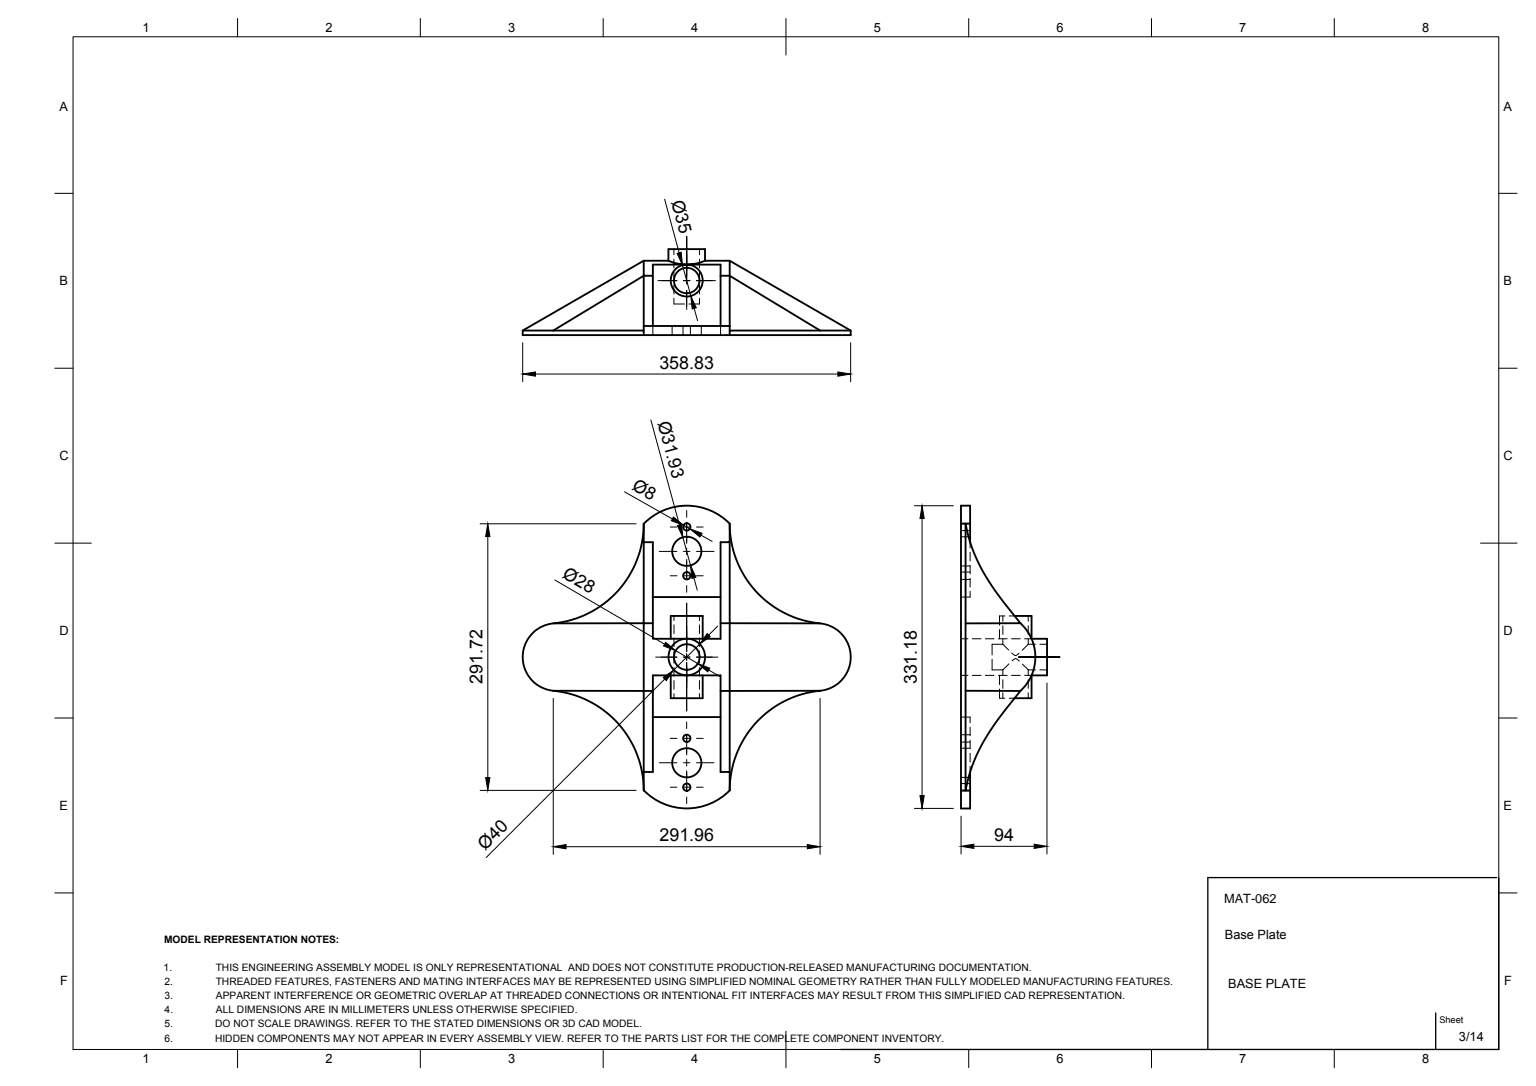
ISO-10303-21;
HEADER;
/* Generated by software containing ST-Developer
 * from STEP Tools, Inc. (www.steptools.com) 
 */

FILE_DESCRIPTION(
/* description */ (''),
/* implementation_level */ '2;1');

FILE_NAME(
/* name */ 'Base Plate.step',
/* time_stamp */ '2026-10-24T10:18:25-07:00',
/* author */ (''),
/* organization */ (''),
/* preprocessor_version */ 'ST-DEVELOPER v20.2',
/* originating_system */ 'Autodesk Translation Framework v15.15.0.0',
/* authorisation */ '');

FILE_SCHEMA (('AUTOMOTIVE_DESIGN { 1 0 10303 214 3 1 1 }'));
ENDSEC;

DATA;
#10=MECHANICAL_DESIGN_GEOMETRIC_PRESENTATION_REPRESENTATION('',(#247),#14125);
#227=SHAPE_REPRESENTATION_RELATIONSHIP('SRR','None',#14200,#237);
#237=ADVANCED_BREP_SHAPE_REPRESENTATION('',(#266),#14114);
#247=STYLED_ITEM('',(#14263),#266);
#266=MANIFOLD_SOLID_BREP('Base Plate',#6134);
#279=B_SPLINE_SURFACE_WITH_KNOTS('',3,1,((#9488,#9489),(#9490,#9491),(#9492,
#9493),(#9494,#9495),(#9496,#9497),(#9498,#9499),(#9500,#9501),(#9502,#9503),
(#9504,#9505),(#9506,#9507),(#9508,#9509),(#9510,#9511),(#9512,#9513),(#9514,
#9515),(#9516,#9517),(#9518,#9519),(#9520,#9521),(#9522,#9523),(#9524,#9525),
(#9526,#9527),(#9528,#9529),(#9530,#9531),(#9532,#9533),(#9534,#9535),(#9536,
#9537),(#9538,#9539),(#9540,#9541),(#9542,#9543),(#9544,#9545),(#9546,#9547)),
 .UNSPECIFIED.,.F.,.F.,.F.,(4,2,2,2,2,2,2,2,2,2,2,2,2,2,4),(2,2),(0.,0.125000000000001,
0.1875,0.25,0.3125,0.375,0.4375,0.5,0.5625,0.625,0.6875,0.75,0.8125,0.875,
1.),(0.,1.00875859451262),.UNSPECIFIED.);
#280=B_SPLINE_SURFACE_WITH_KNOTS('',3,1,((#9560,#9561),(#9562,#9563),(#9564,
#9565),(#9566,#9567),(#9568,#9569),(#9570,#9571),(#9572,#9573),(#9574,#9575),
(#9576,#9577),(#9578,#9579),(#9580,#9581),(#9582,#9583),(#9584,#9585),(#9586,
#9587),(#9588,#9589),(#9590,#9591),(#9592,#9593),(#9594,#9595),(#9596,#9597),
(#9598,#9599),(#9600,#9601),(#9602,#9603),(#9604,#9605),(#9606,#9607),(#9608,
#9609),(#9610,#9611),(#9612,#9613),(#9614,#9615),(#9616,#9617),(#9618,#9619)),
 .UNSPECIFIED.,.F.,.F.,.F.,(4,2,2,2,2,2,2,2,2,2,2,2,2,2,4),(2,2),(0.,0.125,
0.1875,0.25,0.312499999999999,0.374999999999999,0.437499999999999,0.499999999999999,
0.562499999999999,0.624999999999999,0.687499999999999,0.75,0.8125,0.875,
1.),(0.,1.00875859529089),.UNSPECIFIED.);
#281=B_SPLINE_SURFACE_WITH_KNOTS('',3,1,((#9630,#9631),(#9632,#9633),(#9634,
#9635),(#9636,#9637),(#9638,#9639),(#9640,#9641),(#9642,#9643),(#9644,#9645),
(#9646,#9647),(#9648,#9649),(#9650,#9651),(#9652,#9653),(#9654,#9655),(#9656,
#9657),(#9658,#9659),(#9660,#9661),(#9662,#9663),(#9664,#9665),(#9666,#9667),
(#9668,#9669),(#9670,#9671),(#9672,#9673),(#9674,#9675),(#9676,#9677),(#9678,
#9679),(#9680,#9681),(#9682,#9683),(#9684,#9685),(#9686,#9687),(#9688,#9689),
(#9690,#9691),(#9692,#9693),(#9694,#9695),(#9696,#9697)),.UNSPECIFIED.,
 .F.,.F.,.F.,(4,2,2,2,2,2,2,2,2,2,2,2,2,2,2,2,4),(2,2),(0.,0.0625,0.125,
0.1875,0.25,0.3125,0.375,0.4375,0.5,0.5625,0.625,0.6875,0.75,0.8125,0.875,
0.9375,1.),(0.,1.),.UNSPECIFIED.);
#282=B_SPLINE_SURFACE_WITH_KNOTS('',3,1,((#9723,#9724),(#9725,#9726),(#9727,
#9728),(#9729,#9730)),.UNSPECIFIED.,.F.,.F.,.F.,(4,4),(2,2),(0.14457615148808,
1.),(0.,1.2),.UNSPECIFIED.);
#283=B_SPLINE_SURFACE_WITH_KNOTS('',3,1,((#9770,#9771),(#9772,#9773),(#9774,
#9775),(#9776,#9777)),.UNSPECIFIED.,.F.,.F.,.F.,(4,4),(2,2),(0.,0.855423965834485),
(0.,1.2),.UNSPECIFIED.);
#284=B_SPLINE_SURFACE_WITH_KNOTS('',3,1,((#9934,#9935),(#9936,#9937),(#9938,
#9939),(#9940,#9941),(#9942,#9943),(#9944,#9945),(#9946,#9947),(#9948,#9949),
(#9950,#9951),(#9952,#9953),(#9954,#9955),(#9956,#9957),(#9958,#9959),(#9960,
#9961),(#9962,#9963),(#9964,#9965),(#9966,#9967),(#9968,#9969),(#9970,#9971),
(#9972,#9973),(#9974,#9975),(#9976,#9977),(#9978,#9979),(#9980,#9981),(#9982,
#9983),(#9984,#9985),(#9986,#9987),(#9988,#9989),(#9990,#9991),(#9992,#9993)),
 .UNSPECIFIED.,.F.,.F.,.F.,(4,2,2,2,2,2,2,2,2,2,2,2,2,2,4),(2,2),(0.,0.125000000000001,
0.1875,0.25,0.3125,0.375,0.4375,0.5,0.5625,0.625,0.6875,0.75,0.8125,0.875,
1.),(0.,1.00875859388372),.UNSPECIFIED.);
#285=B_SPLINE_SURFACE_WITH_KNOTS('',3,1,((#9999,#10000),(#10001,#10002),
(#10003,#10004),(#10005,#10006),(#10007,#10008),(#10009,#10010),(#10011,
#10012),(#10013,#10014),(#10015,#10016),(#10017,#10018),(#10019,#10020),
(#10021,#10022),(#10023,#10024),(#10025,#10026),(#10027,#10028),(#10029,
#10030),(#10031,#10032),(#10033,#10034),(#10035,#10036),(#10037,#10038),
(#10039,#10040),(#10041,#10042),(#10043,#10044),(#10045,#10046),(#10047,
#10048),(#10049,#10050),(#10051,#10052),(#10053,#10054),(#10055,#10056),
(#10057,#10058)),.UNSPECIFIED.,.F.,.F.,.F.,(4,2,2,2,2,2,2,2,2,2,2,2,2,2,
4),(2,2),(0.,0.125,0.1875,0.25,0.312499999999999,0.374999999999999,0.437499999999999,
0.499999999999999,0.562499999999999,0.624999999999999,0.687499999999999,
0.75,0.8125,0.875,1.),(0.,1.00875859641008),.UNSPECIFIED.);
#286=B_SPLINE_SURFACE_WITH_KNOTS('',3,1,((#10064,#10065),(#10066,#10067),
(#10068,#10069),(#10070,#10071),(#10072,#10073),(#10074,#10075),(#10076,
#10077),(#10078,#10079),(#10080,#10081),(#10082,#10083),(#10084,#10085),
(#10086,#10087),(#10088,#10089),(#10090,#10091),(#10092,#10093),(#10094,
#10095),(#10096,#10097),(#10098,#10099),(#10100,#10101),(#10102,#10103),
(#10104,#10105),(#10106,#10107),(#10108,#10109),(#10110,#10111),(#10112,
#10113),(#10114,#10115),(#10116,#10117),(#10118,#10119),(#10120,#10121),
(#10122,#10123),(#10124,#10125),(#10126,#10127),(#10128,#10129),(#10130,
#10131)),.UNSPECIFIED.,.F.,.F.,.F.,(4,2,2,2,2,2,2,2,2,2,2,2,2,2,2,2,4),
(2,2),(0.,0.0625,0.125,0.1875,0.25,0.3125,0.375,0.4375,0.5,0.5625,0.625,
0.6875,0.75,0.8125,0.875,0.9375,1.),(0.,1.),.UNSPECIFIED.);
#287=B_SPLINE_SURFACE_WITH_KNOTS('',3,1,((#10132,#10133),(#10134,#10135),
(#10136,#10137),(#10138,#10139)),.UNSPECIFIED.,.F.,.F.,.F.,(4,4),(2,2),
(0.144576151499063,1.),(0.,1.20000000000001),.UNSPECIFIED.);
#288=B_SPLINE_SURFACE_WITH_KNOTS('',3,1,((#10140,#10141),(#10142,#10143),
(#10144,#10145),(#10146,#10147)),.UNSPECIFIED.,.F.,.F.,.F.,(4,4),(2,2),
(0.,0.855423965822116),(0.,1.2),.UNSPECIFIED.);
#292=B_SPLINE_CURVE_WITH_KNOTS('',3,(#8671,#8672,#8673,#8674,#8675,#8676,
#8677,#8678,#8679,#8680,#8681,#8682,#8683,#8684,#8685,#8686,#8687,#8688,
#8689,#8690,#8691,#8692,#8693,#8694,#8695,#8696,#8697,#8698,#8699,#8700,
#8701,#8702,#8703,#8704,#8705,#8706,#8707,#8708),.UNSPECIFIED.,.F.,.F.,
(4,2,2,2,2,2,2,2,2,2,2,2,2,2,2,2,2,2,4),(0.,0.0927340025111304,0.185468005022261,
0.370936010044522,0.741872020089043,1.11280803013356,1.48374404017809,2.05783904851561,
2.34488655268438,2.63193405685314,2.9189815610219,3.20602906519066,3.78012407352819,
4.15106008357271,4.52199609361724,4.89293210366176,5.07840010868402,5.17113411119515,
5.26386811370629),.UNSPECIFIED.);
#293=B_SPLINE_CURVE_WITH_KNOTS('',3,(#8709,#8710,#8711,#8712,#8713,#8714,
#8715,#8716,#8717,#8718,#8719,#8720,#8721,#8722,#8723,#8724,#8725,#8726,
#8727,#8728,#8729,#8730,#8731,#8732,#8733,#8734,#8735,#8736,#8737,#8738,
#8739,#8740,#8741,#8742,#8743,#8744,#8745,#8746),.UNSPECIFIED.,.F.,.F.,
(4,2,2,2,2,2,2,2,2,2,2,2,2,2,2,2,2,2,4),(5.26386811370629,5.35660211621742,
5.44933611872855,5.63480412375081,6.00574013379534,6.37667614383986,6.74761215388439,
7.32170716222191,7.60875466639068,7.89580217055944,8.1828496747282,8.46989717889697,
9.0439921872345,9.41492819727902,9.78586420732354,10.1568002173681,10.3422682223903,
10.4350022249015,10.5277362274126),.UNSPECIFIED.);
#294=B_SPLINE_CURVE_WITH_KNOTS('',3,(#8749,#8750,#8751,#8752,#8753,#8754,
#8755,#8756,#8757,#8758,#8759,#8760,#8761,#8762,#8763,#8764,#8765,#8766,
#8767,#8768,#8769,#8770,#8771,#8772,#8773,#8774,#8775,#8776,#8777,#8778,
#8779,#8780,#8781,#8782,#8783,#8784,#8785,#8786),.UNSPECIFIED.,.F.,.F.,
(4,2,2,2,2,2,2,2,2,2,2,2,2,2,2,2,2,2,4),(0.,0.0927340025111308,0.185468005022262,
0.370936010044523,0.741872020089046,1.11280803013357,1.48374404017809,2.05783904851562,
2.34488655268438,2.63193405685315,2.91898156102191,3.20602906519068,3.7801240735282,
4.15106008357273,4.52199609361725,4.89293210366178,5.07840010868404,5.17113411119517,
5.2638681137063),.UNSPECIFIED.);
#295=B_SPLINE_CURVE_WITH_KNOTS('',3,(#8787,#8788,#8789,#8790,#8791,#8792,
#8793,#8794,#8795,#8796,#8797,#8798,#8799,#8800,#8801,#8802,#8803,#8804,
#8805,#8806,#8807,#8808,#8809,#8810,#8811,#8812,#8813,#8814,#8815,#8816,
#8817,#8818,#8819,#8820,#8821,#8822,#8823,#8824),.UNSPECIFIED.,.F.,.F.,
(4,2,2,2,2,2,2,2,2,2,2,2,2,2,2,2,2,2,4),(5.2638681137063,5.35660211621743,
5.44933611872857,5.63480412375083,6.00574013379535,6.37667614383987,6.7476121538844,
7.32170716222192,7.60875466639069,7.89580217055945,8.18284967472821,8.46989717889698,
9.0439921872345,9.41492819727902,9.78586420732355,10.1568002173681,10.3422682223903,
10.4350022249015,10.5277362274126),.UNSPECIFIED.);
#296=B_SPLINE_CURVE_WITH_KNOTS('',3,(#8834,#8835,#8836,#8837,#8838,#8839,
#8840,#8841,#8842,#8843,#8844,#8845,#8846,#8847,#8848,#8849,#8850,#8851),
 .UNSPECIFIED.,.F.,.F.,(4,2,2,2,2,2,2,2,4),(9.15255602234747,9.53372020064684,
9.91488437894621,10.2960485572456,10.6772127355449,11.0587615591079,11.4403103826708,
11.8218592062337,12.2034080297966),.UNSPECIFIED.);
#297=B_SPLINE_CURVE_WITH_KNOTS('',3,(#8853,#8854,#8855,#8856,#8857,#8858,
#8859,#8860,#8861,#8862,#8863,#8864,#8865,#8866,#8867,#8868,#8869,#8870),
 .UNSPECIFIED.,.F.,.F.,(4,2,2,2,2,2,2,2,4),(6.10170401489831,6.48325283846123,
6.86480166202415,7.24635048558707,7.62789930914999,8.00906348744936,8.39022766574873,
8.7713918440481,9.15255602234747),.UNSPECIFIED.);
#298=B_SPLINE_CURVE_WITH_KNOTS('',3,(#8878,#8879,#8880,#8881,#8882,#8883,
#8884,#8885,#8886,#8887,#8888,#8889,#8890,#8891,#8892,#8893,#8894,#8895,
#8896,#8897,#8898,#8899,#8900,#8901,#8902),.UNSPECIFIED.,.F.,.F.,(4,3,3,
3,3,3,3,3,4),(-1.,-0.875,-0.75,-0.625,-0.5,-0.375,-0.25,-0.125,0.),
 .UNSPECIFIED.);
#299=B_SPLINE_CURVE_WITH_KNOTS('',3,(#8935,#8936,#8937,#8938,#8939,#8940,
#8941,#8942,#8943,#8944,#8945,#8946,#8947,#8948,#8949,#8950,#8951,#8952,
#8953,#8954,#8955,#8956,#8957,#8958,#8959,#8960,#8961,#8962,#8963,#8964,
#8965,#8966,#8967,#8968,#8969,#8970,#8971,#8972,#8973,#8974,#8975,#8976,
#8977,#8978,#8979,#8980,#8981,#8982,#8983,#8984,#8985,#8986,#8987,#8988,
#8989,#8990,#8991,#8992,#8993,#8994,#8995,#8996,#8997,#8998,#8999,#9000,
#9001,#9002,#9003,#9004,#9005,#9006,#9007,#9008,#9009,#9010,#9011,#9012,
#9013,#9014,#9015,#9016,#9017,#9018,#9019,#9020,#9021,#9022,#9023,#9024,
#9025,#9026,#9027,#9028,#9029,#9030,#9031,#9032,#9033,#9034,#9035,#9036,
#9037,#9038,#9039,#9040,#9041,#9042,#9043,#9044,#9045,#9046,#9047,#9048,
#9049,#9050,#9051,#9052,#9053,#9054,#9055,#9056,#9057,#9058,#9059,#9060,
#9061,#9062,#9063,#9064,#9065,#9066,#9067,#9068,#9069,#9070,#9071,#9072,
#9073,#9074,#9075,#9076,#9077,#9078,#9079,#9080,#9081,#9082,#9083,#9084,
#9085,#9086,#9087,#9088,#9089,#9090,#9091,#9092,#9093,#9094,#9095,#9096,
#9097,#9098,#9099,#9100,#9101,#9102,#9103,#9104,#9105,#9106,#9107,#9108,
#9109,#9110,#9111,#9112,#9113,#9114,#9115,#9116,#9117,#9118),
 .UNSPECIFIED.,.F.,.F.,(4,3,3,3,3,3,3,3,3,3,3,3,3,3,3,3,3,3,3,3,3,3,3,3,
3,3,3,3,3,3,3,3,3,3,3,3,3,3,3,3,3,3,3,3,3,3,3,3,3,3,3,3,3,3,3,3,3,3,3,3,
3,4),(0.150241198747907,0.167397304835228,0.184718118887321,0.202241047709381,
0.220007464163269,0.238064286953153,0.24996953246951,0.25115288079109,0.277756413628116,
0.304952901732967,0.332851547605054,0.361595243786114,0.371570318101956,
0.374891379875467,0.37684512588001,0.404565053134646,0.433143322897528,
0.46278930680584,0.493811743368577,0.49776633912351,0.499650446210555,0.501139153619483,
0.526262386397414,0.552281259081706,0.580263680389099,0.606497200364781,
0.618794162853381,0.622041027561349,0.623773539268005,0.624868539292833,
0.62607780545653,0.662083917086729,0.720106829170489,0.737600152347333,
0.745800147586479,0.747905908951524,0.749388388026565,0.749955707873429,
0.750554094407055,0.771533017768898,0.793328350135385,0.806245328251924,
0.812300161744051,0.812901601299671,0.828591002192834,0.846067273157757,
0.865308864013037,0.873727060012223,0.874713567355877,0.87499463526931,
0.875252029008748,0.898077041623502,0.91317689673975,0.926104230971432,
0.935341202100003,0.937361789534378,0.937508712583833,0.949516479167898,
0.963001489246603,0.977729187677142,0.995717213427348,1.),.UNSPECIFIED.);
#300=B_SPLINE_CURVE_WITH_KNOTS('',3,(#9125,#9126,#9127,#9128,#9129,#9130,
#9131,#9132,#9133,#9134,#9135,#9136,#9137,#9138,#9139,#9140,#9141,#9142,
#9143,#9144,#9145,#9146,#9147,#9148,#9149,#9150,#9151,#9152,#9153,#9154,
#9155,#9156,#9157,#9158,#9159,#9160,#9161,#9162,#9163,#9164,#9165,#9166,
#9167,#9168,#9169,#9170,#9171,#9172,#9173,#9174,#9175,#9176,#9177,#9178,
#9179,#9180,#9181,#9182,#9183,#9184,#9185,#9186,#9187,#9188,#9189,#9190,
#9191,#9192,#9193,#9194,#9195,#9196,#9197,#9198,#9199,#9200,#9201,#9202,
#9203,#9204,#9205,#9206,#9207,#9208,#9209,#9210,#9211,#9212,#9213,#9214,
#9215,#9216,#9217,#9218,#9219,#9220,#9221,#9222,#9223,#9224,#9225,#9226,
#9227,#9228,#9229,#9230,#9231,#9232,#9233,#9234,#9235,#9236,#9237,#9238,
#9239,#9240,#9241,#9242,#9243,#9244,#9245,#9246,#9247,#9248,#9249,#9250,
#9251,#9252,#9253,#9254,#9255,#9256,#9257,#9258,#9259,#9260,#9261,#9262,
#9263,#9264,#9265,#9266,#9267,#9268,#9269,#9270,#9271,#9272,#9273,#9274,
#9275,#9276,#9277,#9278,#9279,#9280,#9281,#9282,#9283,#9284,#9285,#9286,
#9287,#9288,#9289,#9290,#9291,#9292,#9293,#9294,#9295,#9296,#9297,#9298,
#9299,#9300,#9301,#9302,#9303,#9304,#9305),.UNSPECIFIED.,.F.,.F.,(4,3,3,
3,3,3,3,3,3,3,3,3,3,3,3,3,3,3,3,3,3,3,3,3,3,3,3,3,3,3,3,3,3,3,3,3,3,3,3,
3,3,3,3,3,3,3,3,3,3,3,3,3,3,3,3,3,3,3,3,3,4),(0.,0.0173864418603424,0.0317406407068232,
0.0445735019151384,0.0571545623287322,0.0602506826648901,0.0617926957229375,
0.0622286000993027,0.0624303599347524,0.062594733958677,0.0746665408516836,
0.0885152798747999,0.106661753514485,0.118272684996839,0.12398744033581,
0.12469708287651,0.124978108020046,0.125243557342601,0.14788473893768,0.165674472900084,
0.181276305626835,0.186498845179634,0.187421439977098,0.188081999482287,
0.210113337373066,0.230102338342194,0.249466683031036,0.250074016598888,
0.290650259758732,0.333611006225432,0.365870403860414,0.373431200181113,
0.37495605866907,0.376045195512328,0.405652456316879,0.433409263321146,
0.459431269887646,0.483826901043739,0.495262353148158,0.498872802540326,
0.501065640438556,0.531952057906504,0.561479569871501,0.589959832895018,
0.617600948986098,0.624836289376345,0.626872446293665,0.655342990004338,
0.683068491132681,0.710166098531947,0.73672700441613,0.743791652164193,
0.747103205796098,0.748975108318689,0.750181999132194,0.768352317329036,
0.786243445752231,0.803790273865076,0.82117579398772,0.838357975229974,
0.849761368385144),.UNSPECIFIED.);
#301=B_SPLINE_CURVE_WITH_KNOTS('',3,(#9309,#9310,#9311,#9312),
 .UNSPECIFIED.,.F.,.F.,(4,4),(0.149678083001057,0.999999081493329),
 .UNSPECIFIED.);
#302=B_SPLINE_CURVE_WITH_KNOTS('',3,(#9316,#9317,#9318,#9319),
 .UNSPECIFIED.,.F.,.F.,(4,4),(1.03512807303671E-6,0.850322033620394),
 .UNSPECIFIED.);
#303=B_SPLINE_CURVE_WITH_KNOTS('',3,(#9322,#9323,#9324,#9325),
 .UNSPECIFIED.,.F.,.F.,(4,4),(-1.,-0.850320998496977),.UNSPECIFIED.);
#304=B_SPLINE_CURVE_WITH_KNOTS('',3,(#9330,#9331,#9332,#9333,#9334,#9335),
 .UNSPECIFIED.,.F.,.F.,(4,2,4),(0.,0.125000000000001,0.149679001503013),
 .UNSPECIFIED.);
#305=B_SPLINE_CURVE_WITH_KNOTS('',3,(#9339,#9340,#9341,#9342,#9343,#9344,
#9345,#9346,#9347,#9348,#9349,#9350,#9351,#9352,#9353,#9354,#9355,#9356,
#9357,#9358,#9359,#9360,#9361,#9362,#9363,#9364,#9365,#9366,#9367,#9368,
#9369,#9370,#9371,#9372,#9373,#9374,#9375,#9376,#9377,#9378,#9379,#9380,
#9381,#9382,#9383,#9384),.UNSPECIFIED.,.F.,.F.,(4,3,3,3,3,3,3,3,3,3,3,3,
3,3,3,4),(-16.2042554582664,-16.1371180260605,-14.2967993206844,-13.2982156828388,
-12.2761212402173,-11.2362598068131,-10.1850784450982,-9.12964303443693,
-8.07313766648818,-7.01663510715248,-5.96496475382742,-4.92301254140941,
-3.89517570042547,-2.88556286360814,-1.89741455218585,0.),.UNSPECIFIED.);
#306=B_SPLINE_CURVE_WITH_KNOTS('',3,(#9390,#9391,#9392,#9393,#9394,#9395,
#9396,#9397,#9398,#9399,#9400,#9401,#9402,#9403,#9404,#9405,#9406,#9407,
#9408,#9409,#9410,#9411,#9412,#9413,#9414,#9415,#9416,#9417,#9418,#9419,
#9420,#9421,#9422,#9423,#9424,#9425,#9426,#9427,#9428,#9429,#9430,#9431,
#9432,#9433,#9434,#9435),.UNSPECIFIED.,.F.,.F.,(4,3,3,3,3,3,3,3,3,3,3,3,
3,3,3,4),(-0.0671460795128853,0.,1.84055573902674,2.83926799475898,3.86149408346386,
4.90148945134311,5.95280620554087,7.00837755660534,8.06501900276707,9.12165763995372,
10.1734634487402,11.2155498649205,12.2435190916037,13.2532619668624,14.2415375520883,
16.1391964918471),.UNSPECIFIED.);
#307=B_SPLINE_CURVE_WITH_KNOTS('',3,(#9439,#9440,#9441,#9442,#9443,#9444,
#9445,#9446,#9447,#9448,#9449,#9450,#9451,#9452,#9453,#9454,#9455,#9456,
#9457,#9458,#9459,#9460,#9461,#9462,#9463,#9464,#9465,#9466,#9467,#9468,
#9469,#9470,#9471,#9472,#9473,#9474,#9475,#9476,#9477,#9478,#9479,#9480,
#9481,#9482,#9483,#9484,#9485,#9486,#9487),.UNSPECIFIED.,.F.,.F.,(4,3,3,
3,3,3,3,3,3,3,3,3,3,3,3,3,4),(0.,0.0625,0.125,0.1875,0.25,0.3125,0.375,
0.4375,0.5,0.5625,0.625,0.6875,0.75,0.8125,0.875,0.9375,1.),
 .UNSPECIFIED.);
#308=B_SPLINE_CURVE_WITH_KNOTS('',3,(#9549,#9550,#9551,#9552),
 .UNSPECIFIED.,.F.,.F.,(4,4),(-1.,-0.149679001507915),.UNSPECIFIED.);
#309=B_SPLINE_CURVE_WITH_KNOTS('',3,(#9554,#9555,#9556,#9557,#9558,#9559),
 .UNSPECIFIED.,.F.,.F.,(4,2,4),(0.,0.125000000000001,0.149679001507905),
 .UNSPECIFIED.);
#310=B_SPLINE_CURVE_WITH_KNOTS('',3,(#9620,#9621,#9622,#9623),
 .UNSPECIFIED.,.F.,.F.,(4,4),(-1.,-0.850320998492047),.UNSPECIFIED.);
#311=B_SPLINE_CURVE_WITH_KNOTS('',3,(#9626,#9627,#9628,#9629),
 .UNSPECIFIED.,.F.,.F.,(4,4),(-0.850320998492047,0.),.UNSPECIFIED.);
#312=B_SPLINE_CURVE_WITH_KNOTS('',3,(#9698,#9699,#9700,#9701,#9702,#9703,
#9704,#9705,#9706,#9707,#9708,#9709,#9710,#9711,#9712,#9713,#9714,#9715,
#9716,#9717,#9718,#9719,#9720,#9721,#9722),.UNSPECIFIED.,.F.,.F.,(4,3,3,
3,3,3,3,3,4),(-1.,-0.875,-0.75,-0.625,-0.5,-0.375,-0.25,-0.125,0.),
 .UNSPECIFIED.);
#313=B_SPLINE_CURVE_WITH_KNOTS('',3,(#9734,#9735,#9736,#9737,#9738,#9739,
#9740,#9741,#9742,#9743,#9744,#9745,#9746,#9747,#9748,#9749,#9750,#9751,
#9752,#9753,#9754,#9755,#9756,#9757,#9758,#9759,#9760,#9761,#9762,#9763,
#9764,#9765,#9766,#9767),.UNSPECIFIED.,.F.,.F.,(4,2,2,2,2,2,2,2,2,2,2,2,
2,2,2,2,4),(0.,0.38154882356292,0.76309764712584,1.14464647068876,1.52619529425168,
1.90735947255105,2.28852365085042,2.66968782914979,3.05085200744916,3.43201618574853,
3.8131803640479,4.19434454234727,4.57550872064664,4.95705754420956,5.33860636777248,
5.72015519133539,6.10170401489832),.UNSPECIFIED.);
#314=B_SPLINE_CURVE_WITH_KNOTS('',3,(#9788,#9789,#9790,#9791,#9792,#9793,
#9794,#9795,#9796,#9797,#9798,#9799,#9800,#9801,#9802,#9803,#9804,#9805,
#9806,#9807,#9808,#9809,#9810,#9811,#9812,#9813,#9814,#9815,#9816,#9817,
#9818,#9819,#9820,#9821,#9822,#9823,#9824,#9825,#9826,#9827,#9828,#9829,
#9830,#9831,#9832,#9833),.UNSPECIFIED.,.F.,.F.,(4,3,3,3,3,3,3,3,3,3,3,3,
3,3,3,4),(-16.2042554581874,-16.1371180259159,-14.2967993206444,-13.2982156828138,
-12.2761212402042,-11.2362598068085,-10.1850784450988,-9.12964303443895,
-8.07313766648923,-7.01663510715275,-5.96496475382618,-4.92301254140818,
-3.89517570042437,-2.88556286360765,-1.89741455218581,0.),.UNSPECIFIED.);
#315=B_SPLINE_CURVE_WITH_KNOTS('',3,(#9837,#9838,#9839,#9840,#9841,#9842,
#9843,#9844,#9845,#9846,#9847,#9848,#9849,#9850,#9851,#9852,#9853,#9854,
#9855,#9856,#9857,#9858,#9859,#9860,#9861,#9862,#9863,#9864,#9865,#9866,
#9867,#9868,#9869,#9870,#9871,#9872,#9873,#9874,#9875,#9876,#9877,#9878,
#9879,#9880,#9881,#9882),.UNSPECIFIED.,.F.,.F.,(4,3,3,3,3,3,3,3,3,3,3,3,
3,3,3,4),(-0.0671460794643839,0.,1.84055573907213,2.83926799479983,3.86149408349817,
4.9014894513689,5.95280620555617,7.00837755660805,8.06501900275524,9.12165763992751,
10.1734634486996,11.215549864865,12.2435190915338,13.2532619667787,14.2415375519915,
16.1391964917245),.UNSPECIFIED.);
#316=B_SPLINE_CURVE_WITH_KNOTS('',3,(#9885,#9886,#9887,#9888,#9889,#9890,
#9891,#9892,#9893,#9894,#9895,#9896,#9897,#9898,#9899,#9900,#9901,#9902,
#9903,#9904,#9905,#9906,#9907,#9908,#9909,#9910,#9911,#9912,#9913,#9914,
#9915,#9916,#9917,#9918,#9919,#9920,#9921,#9922,#9923,#9924,#9925,#9926,
#9927,#9928,#9929,#9930,#9931,#9932,#9933),.UNSPECIFIED.,.F.,.F.,(4,3,3,
3,3,3,3,3,3,3,3,3,3,3,3,3,4),(0.,0.0625,0.125,0.1875,0.25,0.3125,0.375,
0.4375,0.5,0.5625,0.625,0.6875,0.75,0.8125,0.875,0.9375,1.),
 .UNSPECIFIED.);
#317=B_SPLINE_CURVE_WITH_KNOTS('',3,(#9994,#9995,#9996,#9997),
 .UNSPECIFIED.,.F.,.F.,(4,4),(-1.,-0.149679001503023),.UNSPECIFIED.);
#318=B_SPLINE_CURVE_WITH_KNOTS('',3,(#10059,#10060,#10061,#10062),
 .UNSPECIFIED.,.F.,.F.,(4,4),(-0.850320998496977,0.),.UNSPECIFIED.);
#477=CYLINDRICAL_SURFACE('',#6280,14.);
#478=CYLINDRICAL_SURFACE('',#6283,13.897506768291);
#479=CYLINDRICAL_SURFACE('',#6285,50.0401279512714);
#480=CYLINDRICAL_SURFACE('',#6301,109.542028553823);
#481=CYLINDRICAL_SURFACE('',#6302,109.542028553823);
#482=CYLINDRICAL_SURFACE('',#6303,37.);
#483=CYLINDRICAL_SURFACE('',#6304,50.0401279512714);
#484=CYLINDRICAL_SURFACE('',#6307,65.8399949356644);
#485=CYLINDRICAL_SURFACE('',#6308,65.8399949356645);
#486=CYLINDRICAL_SURFACE('',#6309,109.542028553823);
#487=CYLINDRICAL_SURFACE('',#6310,109.542028553823);
#488=CYLINDRICAL_SURFACE('',#6311,37.);
#489=CYLINDRICAL_SURFACE('',#6318,17.5);
#490=CYLINDRICAL_SURFACE('',#6322,17.5);
#491=CYLINDRICAL_SURFACE('',#6325,13.897506768291);
#492=CYLINDRICAL_SURFACE('',#6328,20.);
#493=CYLINDRICAL_SURFACE('',#6332,3.99999999999999);
#494=CYLINDRICAL_SURFACE('',#6333,15.9631510575949);
#495=CYLINDRICAL_SURFACE('',#6334,3.99999999999999);
#496=CYLINDRICAL_SURFACE('',#6335,3.99999999999999);
#497=CYLINDRICAL_SURFACE('',#6336,15.9631510575949);
#498=CYLINDRICAL_SURFACE('',#6337,3.99999999999999);
#627=FACE_BOUND('',#1086,.T.);
#628=FACE_BOUND('',#1087,.T.);
#629=FACE_BOUND('',#1088,.T.);
#630=FACE_BOUND('',#1090,.T.);
#631=FACE_BOUND('',#1091,.T.);
#632=FACE_BOUND('',#1092,.T.);
#633=FACE_BOUND('',#1093,.T.);
#634=FACE_BOUND('',#1094,.T.);
#635=FACE_BOUND('',#1095,.T.);
#636=FACE_BOUND('',#1096,.T.);
#637=FACE_BOUND('',#1097,.T.);
#638=FACE_BOUND('',#1099,.T.);
#639=FACE_BOUND('',#1100,.T.);
#640=FACE_BOUND('',#1104,.T.);
#641=FACE_BOUND('',#1105,.T.);
#642=FACE_BOUND('',#1106,.T.);
#643=FACE_BOUND('',#1138,.T.);
#644=FACE_BOUND('',#1141,.T.);
#645=FACE_BOUND('',#1144,.T.);
#732=FACE_OUTER_BOUND('',#1085,.T.);
#733=FACE_OUTER_BOUND('',#1089,.T.);
#734=FACE_OUTER_BOUND('',#1098,.T.);
#735=FACE_OUTER_BOUND('',#1101,.T.);
#736=FACE_OUTER_BOUND('',#1102,.T.);
#737=FACE_OUTER_BOUND('',#1103,.T.);
#738=FACE_OUTER_BOUND('',#1107,.T.);
#739=FACE_OUTER_BOUND('',#1108,.T.);
#740=FACE_OUTER_BOUND('',#1109,.T.);
#741=FACE_OUTER_BOUND('',#1110,.T.);
#742=FACE_OUTER_BOUND('',#1111,.T.);
#743=FACE_OUTER_BOUND('',#1112,.T.);
#744=FACE_OUTER_BOUND('',#1113,.T.);
#745=FACE_OUTER_BOUND('',#1114,.T.);
#746=FACE_OUTER_BOUND('',#1115,.T.);
#747=FACE_OUTER_BOUND('',#1116,.T.);
#748=FACE_OUTER_BOUND('',#1117,.T.);
#749=FACE_OUTER_BOUND('',#1118,.T.);
#750=FACE_OUTER_BOUND('',#1119,.T.);
#751=FACE_OUTER_BOUND('',#1120,.T.);
#752=FACE_OUTER_BOUND('',#1121,.T.);
#753=FACE_OUTER_BOUND('',#1122,.T.);
#754=FACE_OUTER_BOUND('',#1123,.T.);
#755=FACE_OUTER_BOUND('',#1124,.T.);
#756=FACE_OUTER_BOUND('',#1125,.T.);
#757=FACE_OUTER_BOUND('',#1126,.T.);
#758=FACE_OUTER_BOUND('',#1127,.T.);
#759=FACE_OUTER_BOUND('',#1128,.T.);
#760=FACE_OUTER_BOUND('',#1129,.T.);
#761=FACE_OUTER_BOUND('',#1130,.T.);
#762=FACE_OUTER_BOUND('',#1131,.T.);
#763=FACE_OUTER_BOUND('',#1132,.T.);
#764=FACE_OUTER_BOUND('',#1133,.T.);
#765=FACE_OUTER_BOUND('',#1134,.T.);
#766=FACE_OUTER_BOUND('',#1135,.T.);
#767=FACE_OUTER_BOUND('',#1136,.T.);
#768=FACE_OUTER_BOUND('',#1137,.T.);
#769=FACE_OUTER_BOUND('',#1139,.T.);
#770=FACE_OUTER_BOUND('',#1140,.T.);
#771=FACE_OUTER_BOUND('',#1142,.T.);
#772=FACE_OUTER_BOUND('',#1143,.T.);
#773=FACE_OUTER_BOUND('',#1145,.T.);
#774=FACE_OUTER_BOUND('',#1146,.T.);
#775=FACE_OUTER_BOUND('',#1147,.T.);
#776=FACE_OUTER_BOUND('',#1148,.T.);
#777=FACE_OUTER_BOUND('',#1149,.T.);
#778=FACE_OUTER_BOUND('',#1150,.T.);
#779=FACE_OUTER_BOUND('',#1151,.T.);
#780=FACE_OUTER_BOUND('',#1152,.T.);
#781=FACE_OUTER_BOUND('',#1153,.T.);
#782=FACE_OUTER_BOUND('',#1154,.T.);
#1085=EDGE_LOOP('',(#3961,#3962,#3963,#3964,#3965,#3966,#3967,#3968));
#1086=EDGE_LOOP('',(#3969));
#1087=EDGE_LOOP('',(#3970));
#1088=EDGE_LOOP('',(#3971));
#1089=EDGE_LOOP('',(#3972,#3973,#3974,#3975,#3976,#3977,#3978,#3979));
#1090=EDGE_LOOP('',(#3980,#3981,#3982,#3983));
#1091=EDGE_LOOP('',(#3984));
#1092=EDGE_LOOP('',(#3985));
#1093=EDGE_LOOP('',(#3986));
#1094=EDGE_LOOP('',(#3987));
#1095=EDGE_LOOP('',(#3988));
#1096=EDGE_LOOP('',(#3989));
#1097=EDGE_LOOP('',(#3990,#3991,#3992,#3993));
#1098=EDGE_LOOP('',(#3994,#3995,#3996,#3997));
#1099=EDGE_LOOP('',(#3998,#3999));
#1100=EDGE_LOOP('',(#4000,#4001));
#1101=EDGE_LOOP('',(#4002,#4003,#4004,#4005,#4006));
#1102=EDGE_LOOP('',(#4007,#4008,#4009,#4010,#4011,#4012,#4013,#4014,#4015));
#1103=EDGE_LOOP('',(#4016,#4017,#4018,#4019,#4020,#4021,#4022,#4023));
#1104=EDGE_LOOP('',(#4024));
#1105=EDGE_LOOP('',(#4025));
#1106=EDGE_LOOP('',(#4026));
#1107=EDGE_LOOP('',(#4027,#4028,#4029,#4030,#4031,#4032));
#1108=EDGE_LOOP('',(#4033,#4034,#4035,#4036,#4037,#4038));
#1109=EDGE_LOOP('',(#4039,#4040,#4041,#4042,#4043,#4044));
#1110=EDGE_LOOP('',(#4045,#4046,#4047,#4048,#4049,#4050));
#1111=EDGE_LOOP('',(#4051,#4052,#4053));
#1112=EDGE_LOOP('',(#4054,#4055,#4056));
#1113=EDGE_LOOP('',(#4057,#4058,#4059,#4060));
#1114=EDGE_LOOP('',(#4061,#4062,#4063,#4064));
#1115=EDGE_LOOP('',(#4065,#4066,#4067,#4068));
#1116=EDGE_LOOP('',(#4069,#4070,#4071,#4072));
#1117=EDGE_LOOP('',(#4073,#4074,#4075,#4076));
#1118=EDGE_LOOP('',(#4077,#4078,#4079,#4080));
#1119=EDGE_LOOP('',(#4081,#4082,#4083,#4084));
#1120=EDGE_LOOP('',(#4085,#4086,#4087,#4088,#4089,#4090,#4091,#4092));
#1121=EDGE_LOOP('',(#4093,#4094,#4095,#4096));
#1122=EDGE_LOOP('',(#4097,#4098,#4099));
#1123=EDGE_LOOP('',(#4100,#4101,#4102));
#1124=EDGE_LOOP('',(#4103,#4104,#4105,#4106,#4107,#4108));
#1125=EDGE_LOOP('',(#4109,#4110,#4111,#4112,#4113,#4114));
#1126=EDGE_LOOP('',(#4115,#4116,#4117,#4118));
#1127=EDGE_LOOP('',(#4119,#4120,#4121,#4122));
#1128=EDGE_LOOP('',(#4123,#4124,#4125,#4126));
#1129=EDGE_LOOP('',(#4127,#4128,#4129,#4130));
#1130=EDGE_LOOP('',(#4131,#4132,#4133,#4134));
#1131=EDGE_LOOP('',(#4135,#4136,#4137,#4138));
#1132=EDGE_LOOP('',(#4139,#4140,#4141,#4142));
#1133=EDGE_LOOP('',(#4143,#4144,#4145,#4146));
#1134=EDGE_LOOP('',(#4147,#4148,#4149,#4150,#4151,#4152,#4153));
#1135=EDGE_LOOP('',(#4154,#4155,#4156,#4157,#4158,#4159,#4160));
#1136=EDGE_LOOP('',(#4161,#4162,#4163,#4164,#4165));
#1137=EDGE_LOOP('',(#4166));
#1138=EDGE_LOOP('',(#4167));
#1139=EDGE_LOOP('',(#4168,#4169,#4170,#4171,#4172));
#1140=EDGE_LOOP('',(#4173));
#1141=EDGE_LOOP('',(#4174));
#1142=EDGE_LOOP('',(#4175,#4176,#4177,#4178,#4179));
#1143=EDGE_LOOP('',(#4180));
#1144=EDGE_LOOP('',(#4181));
#1145=EDGE_LOOP('',(#4182,#4183,#4184,#4185,#4186,#4187));
#1146=EDGE_LOOP('',(#4188));
#1147=EDGE_LOOP('',(#4189,#4190,#4191,#4192));
#1148=EDGE_LOOP('',(#4193,#4194,#4195,#4196));
#1149=EDGE_LOOP('',(#4197,#4198,#4199,#4200));
#1150=EDGE_LOOP('',(#4201,#4202,#4203,#4204));
#1151=EDGE_LOOP('',(#4205,#4206,#4207,#4208));
#1152=EDGE_LOOP('',(#4209,#4210,#4211,#4212));
#1153=EDGE_LOOP('',(#4213,#4214,#4215,#4216));
#1154=EDGE_LOOP('',(#4217,#4218,#4219,#4220));
#1543=CIRCLE('',#6261,65.8399949356644);
#1544=CIRCLE('',#6262,3.99999999999999);
#1545=CIRCLE('',#6263,15.9631510575949);
#1546=CIRCLE('',#6264,3.99999999999999);
#1547=CIRCLE('',#6266,109.542028553823);
#1548=CIRCLE('',#6267,65.8399949356645);
#1549=CIRCLE('',#6268,109.542028553823);
#1550=CIRCLE('',#6269,37.);
#1551=CIRCLE('',#6270,109.542028553823);
#1552=CIRCLE('',#6271,65.8399949356644);
#1553=CIRCLE('',#6272,109.542028553823);
#1554=CIRCLE('',#6273,37.);
#1555=CIRCLE('',#6274,3.99999999999999);
#1556=CIRCLE('',#6275,15.9631510575949);
#1557=CIRCLE('',#6276,3.99999999999999);
#1558=CIRCLE('',#6277,3.99999999999999);
#1559=CIRCLE('',#6278,15.9631510575949);
#1560=CIRCLE('',#6279,3.99999999999999);
#1561=CIRCLE('',#6281,14.);
#1562=CIRCLE('',#6282,14.);
#1563=CIRCLE('',#6284,13.897506768291);
#1564=CIRCLE('',#6286,50.0401279512714);
#1565=CIRCLE('',#6287,50.0401279512714);
#1566=CIRCLE('',#6289,65.8399949356645);
#1567=CIRCLE('',#6290,3.99999999999999);
#1568=CIRCLE('',#6291,15.9631510575949);
#1569=CIRCLE('',#6292,3.99999999999999);
#1570=CIRCLE('',#6294,50.0401279512714);
#1571=CIRCLE('',#6296,50.0401279512714);
#1572=CIRCLE('',#6313,17.5);
#1573=CIRCLE('',#6314,17.5);
#1574=CIRCLE('',#6316,17.5);
#1575=CIRCLE('',#6317,17.5);
#1576=CIRCLE('',#6319,17.5);
#1577=CIRCLE('',#6321,13.897506768291);
#1578=CIRCLE('',#6323,17.5);
#1579=CIRCLE('',#6327,20.);
#1803=LINE('',#8598,#2191);
#1804=LINE('',#8600,#2192);
#1805=LINE('',#8602,#2193);
#1806=LINE('',#8604,#2194);
#1807=LINE('',#8606,#2195);
#1808=LINE('',#8610,#2196);
#1809=LINE('',#8611,#2197);
#1810=LINE('',#8637,#2198);
#1811=LINE('',#8639,#2199);
#1812=LINE('',#8641,#2200);
#1813=LINE('',#8642,#2201);
#1814=LINE('',#8657,#2202);
#1815=LINE('',#8659,#2203);
#1816=LINE('',#8661,#2204);
#1817=LINE('',#8662,#2205);
#1818=LINE('',#8667,#2206);
#1819=LINE('',#8828,#2207);
#1820=LINE('',#8832,#2208);
#1821=LINE('',#8872,#2209);
#1822=LINE('',#8876,#2210);
#1823=LINE('',#8904,#2211);
#1824=LINE('',#8909,#2212);
#1825=LINE('',#8911,#2213);
#1826=LINE('',#8913,#2214);
#1827=LINE('',#8915,#2215);
#1828=LINE('',#8919,#2216);
#1829=LINE('',#8921,#2217);
#1830=LINE('',#8922,#2218);
#1831=LINE('',#8933,#2219);
#1832=LINE('',#8934,#2220);
#1833=LINE('',#9120,#2221);
#1834=LINE('',#9122,#2222);
#1835=LINE('',#9307,#2223);
#1836=LINE('',#9308,#2224);
#1837=LINE('',#9314,#2225);
#1838=LINE('',#9315,#2226);
#1839=LINE('',#9326,#2227);
#1840=LINE('',#9329,#2228);
#1841=LINE('',#9385,#2229);
#1842=LINE('',#9386,#2230);
#1843=LINE('',#9436,#2231);
#1844=LINE('',#9437,#2232);
#1845=LINE('',#9553,#2233);
#1846=LINE('',#9625,#2234);
#1847=LINE('',#9731,#2235);
#1848=LINE('',#9733,#2236);
#1849=LINE('',#9768,#2237);
#1850=LINE('',#9769,#2238);
#1851=LINE('',#9779,#2239);
#1852=LINE('',#9781,#2240);
#1853=LINE('',#9783,#2241);
#1854=LINE('',#9785,#2242);
#1855=LINE('',#9834,#2243);
#1856=LINE('',#9883,#2244);
#1857=LINE('',#9998,#2245);
#1858=LINE('',#10063,#2246);
#1859=LINE('',#10158,#2247);
#1860=LINE('',#10165,#2248);
#1861=LINE('',#10169,#2249);
#1862=LINE('',#10174,#2250);
#1863=LINE('',#10179,#2251);
#1864=LINE('',#10181,#2252);
#1865=LINE('',#10183,#2253);
#1866=LINE('',#10185,#2254);
#1867=LINE('',#10187,#2255);
#1868=LINE('',#10189,#2256);
#2191=VECTOR('',#6913,60.0123183146203);
#2192=VECTOR('',#6914,74.);
#2193=VECTOR('',#6915,60.0123183146203);
#2194=VECTOR('',#6916,10.);
#2195=VECTOR('',#6917,20.1794558564032);
#2196=VECTOR('',#6920,20.1794558568838);
#2197=VECTOR('',#6921,10.);
#2198=VECTOR('',#6946,74.);
#2199=VECTOR('',#6947,45.6680057154832);
#2200=VECTOR('',#6948,74.);
#2201=VECTOR('',#6949,45.6680057154831);
#2202=VECTOR('',#6962,45.6680057154832);
#2203=VECTOR('',#6963,74.);
#2204=VECTOR('',#6964,45.6680057154831);
#2205=VECTOR('',#6965,74.);
#2206=VECTOR('',#6970,14.);
#2207=VECTOR('',#6977,13.897506768291);
#2208=VECTOR('',#6980,37.);
#2209=VECTOR('',#6981,37.);
#2210=VECTOR('',#6984,10.);
#2211=VECTOR('',#6985,10.);
#2212=VECTOR('',#6990,74.);
#2213=VECTOR('',#6991,60.0123511269393);
#2214=VECTOR('',#6992,10.);
#2215=VECTOR('',#6993,20.1794558568839);
#2216=VECTOR('',#6996,20.1794558564032);
#2217=VECTOR('',#6997,10.);
#2218=VECTOR('',#6998,60.0123511269481);
#2219=VECTOR('',#7009,77.1122755947453);
#2220=VECTOR('',#7010,10.);
#2221=VECTOR('',#7013,10.);
#2222=VECTOR('',#7014,77.1122755947453);
#2223=VECTOR('',#7019,10.);
#2224=VECTOR('',#7020,77.1122755947453);
#2225=VECTOR('',#7023,77.1122755947453);
#2226=VECTOR('',#7024,10.);
#2227=VECTOR('',#7027,4.99999999999998);
#2228=VECTOR('',#7030,4.99999999999998);
#2229=VECTOR('',#7033,5.);
#2230=VECTOR('',#7034,5.);
#2231=VECTOR('',#7037,5.);
#2232=VECTOR('',#7038,5.);
#2233=VECTOR('',#7041,10.);
#2234=VECTOR('',#7042,10.);
#2235=VECTOR('',#7043,10.);
#2236=VECTOR('',#7046,37.);
#2237=VECTOR('',#7047,37.);
#2238=VECTOR('',#7048,10.);
#2239=VECTOR('',#7051,5.);
#2240=VECTOR('',#7054,5.);
#2241=VECTOR('',#7057,5.00000000000002);
#2242=VECTOR('',#7060,5.00000000000002);
#2243=VECTOR('',#7063,5.);
#2244=VECTOR('',#7066,5.);
#2245=VECTOR('',#7069,10.);
#2246=VECTOR('',#7070,10.);
#2247=VECTOR('',#7085,17.5);
#2248=VECTOR('',#7094,17.5);
#2249=VECTOR('',#7101,13.897506768291);
#2250=VECTOR('',#7108,20.);
#2251=VECTOR('',#7117,3.99999999999999);
#2252=VECTOR('',#7120,15.9631510575949);
#2253=VECTOR('',#7123,3.99999999999999);
#2254=VECTOR('',#7126,3.99999999999999);
#2255=VECTOR('',#7129,15.9631510575949);
#2256=VECTOR('',#7132,3.99999999999999);
#2579=VERTEX_POINT('',#8596);
#2580=VERTEX_POINT('',#8597);
#2581=VERTEX_POINT('',#8599);
#2582=VERTEX_POINT('',#8601);
#2583=VERTEX_POINT('',#8603);
#2584=VERTEX_POINT('',#8605);
#2585=VERTEX_POINT('',#8607);
#2586=VERTEX_POINT('',#8609);
#2587=VERTEX_POINT('',#8612);
#2588=VERTEX_POINT('',#8614);
#2589=VERTEX_POINT('',#8616);
#2590=VERTEX_POINT('',#8619);
#2591=VERTEX_POINT('',#8620);
#2592=VERTEX_POINT('',#8622);
#2593=VERTEX_POINT('',#8624);
#2594=VERTEX_POINT('',#8626);
#2595=VERTEX_POINT('',#8628);
#2596=VERTEX_POINT('',#8630);
#2597=VERTEX_POINT('',#8632);
#2598=VERTEX_POINT('',#8635);
#2599=VERTEX_POINT('',#8636);
#2600=VERTEX_POINT('',#8638);
#2601=VERTEX_POINT('',#8640);
#2602=VERTEX_POINT('',#8643);
#2603=VERTEX_POINT('',#8645);
#2604=VERTEX_POINT('',#8647);
#2605=VERTEX_POINT('',#8649);
#2606=VERTEX_POINT('',#8651);
#2607=VERTEX_POINT('',#8653);
#2608=VERTEX_POINT('',#8655);
#2609=VERTEX_POINT('',#8656);
#2610=VERTEX_POINT('',#8658);
#2611=VERTEX_POINT('',#8660);
#2612=VERTEX_POINT('',#8664);
#2613=VERTEX_POINT('',#8666);
#2614=VERTEX_POINT('',#8669);
#2615=VERTEX_POINT('',#8670);
#2616=VERTEX_POINT('',#8747);
#2617=VERTEX_POINT('',#8748);
#2618=VERTEX_POINT('',#8826);
#2619=VERTEX_POINT('',#8830);
#2620=VERTEX_POINT('',#8831);
#2621=VERTEX_POINT('',#8833);
#2622=VERTEX_POINT('',#8852);
#2623=VERTEX_POINT('',#8871);
#2624=VERTEX_POINT('',#8873);
#2625=VERTEX_POINT('',#8875);
#2626=VERTEX_POINT('',#8877);
#2627=VERTEX_POINT('',#8903);
#2628=VERTEX_POINT('',#8907);
#2629=VERTEX_POINT('',#8908);
#2630=VERTEX_POINT('',#8910);
#2631=VERTEX_POINT('',#8912);
#2632=VERTEX_POINT('',#8914);
#2633=VERTEX_POINT('',#8916);
#2634=VERTEX_POINT('',#8918);
#2635=VERTEX_POINT('',#8920);
#2636=VERTEX_POINT('',#8923);
#2637=VERTEX_POINT('',#8925);
#2638=VERTEX_POINT('',#8927);
#2639=VERTEX_POINT('',#8930);
#2640=VERTEX_POINT('',#8931);
#2641=VERTEX_POINT('',#9121);
#2642=VERTEX_POINT('',#9123);
#2643=VERTEX_POINT('',#9321);
#2644=VERTEX_POINT('',#9328);
#2645=VERTEX_POINT('',#9337);
#2646=VERTEX_POINT('',#9338);
#2647=VERTEX_POINT('',#9388);
#2648=VERTEX_POINT('',#9389);
#2649=VERTEX_POINT('',#9548);
#2650=VERTEX_POINT('',#9624);
#2651=VERTEX_POINT('',#9787);
#2652=VERTEX_POINT('',#9836);
#2653=VERTEX_POINT('',#10149);
#2654=VERTEX_POINT('',#10153);
#2655=VERTEX_POINT('',#10157);
#2656=VERTEX_POINT('',#10161);
#2657=VERTEX_POINT('',#10164);
#2658=VERTEX_POINT('',#10171);
#3128=EDGE_CURVE('',#2579,#2580,#1803,.T.);
#3129=EDGE_CURVE('',#2580,#2581,#1804,.T.);
#3130=EDGE_CURVE('',#2582,#2581,#1805,.T.);
#3131=EDGE_CURVE('',#2582,#2583,#1806,.T.);
#3132=EDGE_CURVE('',#2583,#2584,#1807,.T.);
#3133=EDGE_CURVE('',#2584,#2585,#1543,.T.);
#3134=EDGE_CURVE('',#2585,#2586,#1808,.T.);
#3135=EDGE_CURVE('',#2579,#2586,#1809,.T.);
#3136=EDGE_CURVE('',#2587,#2587,#1544,.T.);
#3137=EDGE_CURVE('',#2588,#2588,#1545,.T.);
#3138=EDGE_CURVE('',#2589,#2589,#1546,.T.);
#3139=EDGE_CURVE('',#2590,#2591,#1547,.T.);
#3140=EDGE_CURVE('',#2592,#2590,#1548,.T.);
#3141=EDGE_CURVE('',#2592,#2593,#1549,.T.);
#3142=EDGE_CURVE('',#2594,#2593,#1550,.T.);
#3143=EDGE_CURVE('',#2595,#2594,#1551,.T.);
#3144=EDGE_CURVE('',#2596,#2595,#1552,.T.);
#3145=EDGE_CURVE('',#2596,#2597,#1553,.T.);
#3146=EDGE_CURVE('',#2597,#2591,#1554,.T.);
#3147=EDGE_CURVE('',#2598,#2599,#1810,.T.);
#3148=EDGE_CURVE('',#2600,#2598,#1811,.T.);
#3149=EDGE_CURVE('',#2601,#2600,#1812,.T.);
#3150=EDGE_CURVE('',#2599,#2601,#1813,.T.);
#3151=EDGE_CURVE('',#2602,#2602,#1555,.F.);
#3152=EDGE_CURVE('',#2603,#2603,#1556,.F.);
#3153=EDGE_CURVE('',#2604,#2604,#1557,.F.);
#3154=EDGE_CURVE('',#2605,#2605,#1558,.T.);
#3155=EDGE_CURVE('',#2606,#2606,#1559,.T.);
#3156=EDGE_CURVE('',#2607,#2607,#1560,.T.);
#3157=EDGE_CURVE('',#2608,#2609,#1814,.T.);
#3158=EDGE_CURVE('',#2609,#2610,#1815,.T.);
#3159=EDGE_CURVE('',#2610,#2611,#1816,.T.);
#3160=EDGE_CURVE('',#2611,#2608,#1817,.T.);
#3161=EDGE_CURVE('',#2612,#2612,#1561,.F.);
#3162=EDGE_CURVE('',#2612,#2613,#1818,.T.);
#3163=EDGE_CURVE('',#2613,#2613,#1562,.T.);
#3164=EDGE_CURVE('',#2614,#2615,#292,.T.);
#3165=EDGE_CURVE('',#2615,#2614,#293,.T.);
#3166=EDGE_CURVE('',#2616,#2617,#294,.T.);
#3167=EDGE_CURVE('',#2617,#2616,#295,.T.);
#3168=EDGE_CURVE('',#2618,#2618,#1563,.T.);
#3169=EDGE_CURVE('',#2618,#2617,#1819,.T.);
#3170=EDGE_CURVE('',#2619,#2620,#1820,.T.);
#3171=EDGE_CURVE('',#2621,#2620,#296,.T.);
#3172=EDGE_CURVE('',#2622,#2621,#297,.T.);
#3173=EDGE_CURVE('',#2623,#2622,#1821,.T.);
#3174=EDGE_CURVE('',#2623,#2624,#1564,.T.);
#3175=EDGE_CURVE('',#2624,#2625,#1822,.T.);
#3176=EDGE_CURVE('',#2626,#2625,#298,.T.);
#3177=EDGE_CURVE('',#2627,#2626,#1823,.T.);
#3178=EDGE_CURVE('',#2627,#2619,#1565,.T.);
#3179=EDGE_CURVE('',#2628,#2629,#1824,.T.);
#3180=EDGE_CURVE('',#2628,#2630,#1825,.T.);
#3181=EDGE_CURVE('',#2631,#2630,#1826,.F.);
#3182=EDGE_CURVE('',#2631,#2632,#1827,.T.);
#3183=EDGE_CURVE('',#2632,#2633,#1566,.T.);
#3184=EDGE_CURVE('',#2633,#2634,#1828,.T.);
#3185=EDGE_CURVE('',#2634,#2635,#1829,.F.);
#3186=EDGE_CURVE('',#2629,#2635,#1830,.T.);
#3187=EDGE_CURVE('',#2636,#2636,#1567,.T.);
#3188=EDGE_CURVE('',#2637,#2637,#1568,.T.);
#3189=EDGE_CURVE('',#2638,#2638,#1569,.T.);
#3190=EDGE_CURVE('',#2639,#2640,#1570,.T.);
#3191=EDGE_CURVE('',#2599,#2640,#1831,.T.);
#3192=EDGE_CURVE('',#2601,#2580,#1832,.T.);
#3193=EDGE_CURVE('',#2579,#2639,#299,.T.);
#3194=EDGE_CURVE('',#2611,#2628,#1833,.T.);
#3195=EDGE_CURVE('',#2641,#2610,#1834,.T.);
#3196=EDGE_CURVE('',#2641,#2642,#1571,.T.);
#3197=EDGE_CURVE('',#2642,#2630,#300,.T.);
#3198=EDGE_CURVE('',#2600,#2581,#1835,.T.);
#3199=EDGE_CURVE('',#2619,#2598,#1836,.T.);
#3200=EDGE_CURVE('',#2582,#2627,#301,.F.);
#3201=EDGE_CURVE('',#2609,#2623,#1837,.T.);
#3202=EDGE_CURVE('',#2608,#2629,#1838,.T.);
#3203=EDGE_CURVE('',#2624,#2635,#302,.F.);
#3204=EDGE_CURVE('',#2643,#2583,#303,.T.);
#3205=EDGE_CURVE('',#2643,#2584,#1839,.T.);
#3206=EDGE_CURVE('',#2644,#2633,#1840,.T.);
#3207=EDGE_CURVE('',#2644,#2634,#304,.T.);
#3208=EDGE_CURVE('',#2645,#2646,#305,.T.);
#3209=EDGE_CURVE('',#2595,#2645,#1841,.T.);
#3210=EDGE_CURVE('',#2594,#2646,#1842,.T.);
#3211=EDGE_CURVE('',#2647,#2648,#306,.T.);
#3212=EDGE_CURVE('',#2593,#2648,#1843,.T.);
#3213=EDGE_CURVE('',#2592,#2647,#1844,.T.);
#3214=EDGE_CURVE('',#2646,#2648,#307,.T.);
#3215=EDGE_CURVE('',#2649,#2631,#308,.T.);
#3216=EDGE_CURVE('',#2649,#2648,#1845,.T.);
#3217=EDGE_CURVE('',#2647,#2631,#309,.T.);
#3218=EDGE_CURVE('',#2645,#2586,#310,.T.);
#3219=EDGE_CURVE('',#2646,#2650,#1846,.T.);
#3220=EDGE_CURVE('',#2586,#2650,#311,.T.);
#3221=EDGE_CURVE('',#2650,#2649,#312,.T.);
#3222=EDGE_CURVE('',#2639,#2650,#1847,.T.);
#3223=EDGE_CURVE('',#2622,#2641,#1848,.T.);
#3224=EDGE_CURVE('',#2620,#2622,#313,.T.);
#3225=EDGE_CURVE('',#2620,#2640,#1849,.T.);
#3226=EDGE_CURVE('',#2642,#2649,#1850,.T.);
#3227=EDGE_CURVE('',#2645,#2585,#1851,.T.);
#3228=EDGE_CURVE('',#2647,#2632,#1852,.T.);
#3229=EDGE_CURVE('',#2596,#2643,#1853,.T.);
#3230=EDGE_CURVE('',#2590,#2644,#1854,.T.);
#3231=EDGE_CURVE('',#2643,#2651,#314,.T.);
#3232=EDGE_CURVE('',#2597,#2651,#1855,.T.);
#3233=EDGE_CURVE('',#2644,#2652,#315,.T.);
#3234=EDGE_CURVE('',#2591,#2652,#1856,.T.);
#3235=EDGE_CURVE('',#2651,#2652,#316,.T.);
#3236=EDGE_CURVE('',#2625,#2634,#317,.T.);
#3237=EDGE_CURVE('',#2625,#2652,#1857,.T.);
#3238=EDGE_CURVE('',#2583,#2626,#318,.T.);
#3239=EDGE_CURVE('',#2651,#2626,#1858,.T.);
#3240=EDGE_CURVE('',#2653,#2620,#1572,.T.);
#3241=EDGE_CURVE('',#2620,#2653,#1573,.T.);
#3242=EDGE_CURVE('',#2622,#2654,#1574,.T.);
#3243=EDGE_CURVE('',#2654,#2622,#1575,.T.);
#3244=EDGE_CURVE('',#2653,#2655,#1859,.T.);
#3245=EDGE_CURVE('',#2655,#2655,#1576,.T.);
#3246=EDGE_CURVE('',#2656,#2656,#1577,.T.);
#3247=EDGE_CURVE('',#2654,#2657,#1860,.T.);
#3248=EDGE_CURVE('',#2657,#2657,#1578,.T.);
#3249=EDGE_CURVE('',#2615,#2656,#1861,.T.);
#3250=EDGE_CURVE('',#2658,#2658,#1579,.T.);
#3251=EDGE_CURVE('',#2658,#2621,#1862,.T.);
#3252=EDGE_CURVE('',#2607,#2589,#1863,.T.);
#3253=EDGE_CURVE('',#2606,#2588,#1864,.T.);
#3254=EDGE_CURVE('',#2605,#2587,#1865,.T.);
#3255=EDGE_CURVE('',#2604,#2638,#1866,.T.);
#3256=EDGE_CURVE('',#2603,#2637,#1867,.T.);
#3257=EDGE_CURVE('',#2602,#2636,#1868,.T.);
#3961=ORIENTED_EDGE('',*,*,#3128,.T.);
#3962=ORIENTED_EDGE('',*,*,#3129,.T.);
#3963=ORIENTED_EDGE('',*,*,#3130,.F.);
#3964=ORIENTED_EDGE('',*,*,#3131,.T.);
#3965=ORIENTED_EDGE('',*,*,#3132,.T.);
#3966=ORIENTED_EDGE('',*,*,#3133,.T.);
#3967=ORIENTED_EDGE('',*,*,#3134,.T.);
#3968=ORIENTED_EDGE('',*,*,#3135,.F.);
#3969=ORIENTED_EDGE('',*,*,#3136,.F.);
#3970=ORIENTED_EDGE('',*,*,#3137,.F.);
#3971=ORIENTED_EDGE('',*,*,#3138,.F.);
#3972=ORIENTED_EDGE('',*,*,#3139,.F.);
#3973=ORIENTED_EDGE('',*,*,#3140,.F.);
#3974=ORIENTED_EDGE('',*,*,#3141,.T.);
#3975=ORIENTED_EDGE('',*,*,#3142,.F.);
#3976=ORIENTED_EDGE('',*,*,#3143,.F.);
#3977=ORIENTED_EDGE('',*,*,#3144,.F.);
#3978=ORIENTED_EDGE('',*,*,#3145,.T.);
#3979=ORIENTED_EDGE('',*,*,#3146,.T.);
#3980=ORIENTED_EDGE('',*,*,#3147,.F.);
#3981=ORIENTED_EDGE('',*,*,#3148,.F.);
#3982=ORIENTED_EDGE('',*,*,#3149,.F.);
#3983=ORIENTED_EDGE('',*,*,#3150,.F.);
#3984=ORIENTED_EDGE('',*,*,#3151,.T.);
#3985=ORIENTED_EDGE('',*,*,#3152,.T.);
#3986=ORIENTED_EDGE('',*,*,#3153,.T.);
#3987=ORIENTED_EDGE('',*,*,#3154,.F.);
#3988=ORIENTED_EDGE('',*,*,#3155,.F.);
#3989=ORIENTED_EDGE('',*,*,#3156,.F.);
#3990=ORIENTED_EDGE('',*,*,#3157,.T.);
#3991=ORIENTED_EDGE('',*,*,#3158,.T.);
#3992=ORIENTED_EDGE('',*,*,#3159,.T.);
#3993=ORIENTED_EDGE('',*,*,#3160,.T.);
#3994=ORIENTED_EDGE('',*,*,#3161,.F.);
#3995=ORIENTED_EDGE('',*,*,#3162,.T.);
#3996=ORIENTED_EDGE('',*,*,#3163,.T.);
#3997=ORIENTED_EDGE('',*,*,#3162,.F.);
#3998=ORIENTED_EDGE('',*,*,#3164,.T.);
#3999=ORIENTED_EDGE('',*,*,#3165,.T.);
#4000=ORIENTED_EDGE('',*,*,#3166,.T.);
#4001=ORIENTED_EDGE('',*,*,#3167,.T.);
#4002=ORIENTED_EDGE('',*,*,#3168,.T.);
#4003=ORIENTED_EDGE('',*,*,#3169,.T.);
#4004=ORIENTED_EDGE('',*,*,#3166,.F.);
#4005=ORIENTED_EDGE('',*,*,#3167,.F.);
#4006=ORIENTED_EDGE('',*,*,#3169,.F.);
#4007=ORIENTED_EDGE('',*,*,#3170,.T.);
#4008=ORIENTED_EDGE('',*,*,#3171,.F.);
#4009=ORIENTED_EDGE('',*,*,#3172,.F.);
#4010=ORIENTED_EDGE('',*,*,#3173,.F.);
#4011=ORIENTED_EDGE('',*,*,#3174,.T.);
#4012=ORIENTED_EDGE('',*,*,#3175,.T.);
#4013=ORIENTED_EDGE('',*,*,#3176,.F.);
#4014=ORIENTED_EDGE('',*,*,#3177,.F.);
#4015=ORIENTED_EDGE('',*,*,#3178,.T.);
#4016=ORIENTED_EDGE('',*,*,#3179,.F.);
#4017=ORIENTED_EDGE('',*,*,#3180,.T.);
#4018=ORIENTED_EDGE('',*,*,#3181,.F.);
#4019=ORIENTED_EDGE('',*,*,#3182,.T.);
#4020=ORIENTED_EDGE('',*,*,#3183,.T.);
#4021=ORIENTED_EDGE('',*,*,#3184,.T.);
#4022=ORIENTED_EDGE('',*,*,#3185,.T.);
#4023=ORIENTED_EDGE('',*,*,#3186,.F.);
#4024=ORIENTED_EDGE('',*,*,#3187,.T.);
#4025=ORIENTED_EDGE('',*,*,#3188,.T.);
#4026=ORIENTED_EDGE('',*,*,#3189,.T.);
#4027=ORIENTED_EDGE('',*,*,#3190,.T.);
#4028=ORIENTED_EDGE('',*,*,#3191,.F.);
#4029=ORIENTED_EDGE('',*,*,#3150,.T.);
#4030=ORIENTED_EDGE('',*,*,#3192,.T.);
#4031=ORIENTED_EDGE('',*,*,#3128,.F.);
#4032=ORIENTED_EDGE('',*,*,#3193,.T.);
#4033=ORIENTED_EDGE('',*,*,#3180,.F.);
#4034=ORIENTED_EDGE('',*,*,#3194,.F.);
#4035=ORIENTED_EDGE('',*,*,#3159,.F.);
#4036=ORIENTED_EDGE('',*,*,#3195,.F.);
#4037=ORIENTED_EDGE('',*,*,#3196,.T.);
#4038=ORIENTED_EDGE('',*,*,#3197,.T.);
#4039=ORIENTED_EDGE('',*,*,#3130,.T.);
#4040=ORIENTED_EDGE('',*,*,#3198,.F.);
#4041=ORIENTED_EDGE('',*,*,#3148,.T.);
#4042=ORIENTED_EDGE('',*,*,#3199,.F.);
#4043=ORIENTED_EDGE('',*,*,#3178,.F.);
#4044=ORIENTED_EDGE('',*,*,#3200,.F.);
#4045=ORIENTED_EDGE('',*,*,#3174,.F.);
#4046=ORIENTED_EDGE('',*,*,#3201,.F.);
#4047=ORIENTED_EDGE('',*,*,#3157,.F.);
#4048=ORIENTED_EDGE('',*,*,#3202,.T.);
#4049=ORIENTED_EDGE('',*,*,#3186,.T.);
#4050=ORIENTED_EDGE('',*,*,#3203,.F.);
#4051=ORIENTED_EDGE('',*,*,#3132,.F.);
#4052=ORIENTED_EDGE('',*,*,#3204,.F.);
#4053=ORIENTED_EDGE('',*,*,#3205,.T.);
#4054=ORIENTED_EDGE('',*,*,#3206,.F.);
#4055=ORIENTED_EDGE('',*,*,#3207,.T.);
#4056=ORIENTED_EDGE('',*,*,#3184,.F.);
#4057=ORIENTED_EDGE('',*,*,#3208,.F.);
#4058=ORIENTED_EDGE('',*,*,#3209,.F.);
#4059=ORIENTED_EDGE('',*,*,#3143,.T.);
#4060=ORIENTED_EDGE('',*,*,#3210,.T.);
#4061=ORIENTED_EDGE('',*,*,#3211,.T.);
#4062=ORIENTED_EDGE('',*,*,#3212,.F.);
#4063=ORIENTED_EDGE('',*,*,#3141,.F.);
#4064=ORIENTED_EDGE('',*,*,#3213,.T.);
#4065=ORIENTED_EDGE('',*,*,#3214,.F.);
#4066=ORIENTED_EDGE('',*,*,#3210,.F.);
#4067=ORIENTED_EDGE('',*,*,#3142,.T.);
#4068=ORIENTED_EDGE('',*,*,#3212,.T.);
#4069=ORIENTED_EDGE('',*,*,#3215,.F.);
#4070=ORIENTED_EDGE('',*,*,#3216,.T.);
#4071=ORIENTED_EDGE('',*,*,#3211,.F.);
#4072=ORIENTED_EDGE('',*,*,#3217,.T.);
#4073=ORIENTED_EDGE('',*,*,#3218,.F.);
#4074=ORIENTED_EDGE('',*,*,#3208,.T.);
#4075=ORIENTED_EDGE('',*,*,#3219,.T.);
#4076=ORIENTED_EDGE('',*,*,#3220,.F.);
#4077=ORIENTED_EDGE('',*,*,#3221,.F.);
#4078=ORIENTED_EDGE('',*,*,#3219,.F.);
#4079=ORIENTED_EDGE('',*,*,#3214,.T.);
#4080=ORIENTED_EDGE('',*,*,#3216,.F.);
#4081=ORIENTED_EDGE('',*,*,#3193,.F.);
#4082=ORIENTED_EDGE('',*,*,#3135,.T.);
#4083=ORIENTED_EDGE('',*,*,#3220,.T.);
#4084=ORIENTED_EDGE('',*,*,#3222,.F.);
#4085=ORIENTED_EDGE('',*,*,#3223,.F.);
#4086=ORIENTED_EDGE('',*,*,#3224,.F.);
#4087=ORIENTED_EDGE('',*,*,#3225,.T.);
#4088=ORIENTED_EDGE('',*,*,#3190,.F.);
#4089=ORIENTED_EDGE('',*,*,#3222,.T.);
#4090=ORIENTED_EDGE('',*,*,#3221,.T.);
#4091=ORIENTED_EDGE('',*,*,#3226,.F.);
#4092=ORIENTED_EDGE('',*,*,#3196,.F.);
#4093=ORIENTED_EDGE('',*,*,#3215,.T.);
#4094=ORIENTED_EDGE('',*,*,#3181,.T.);
#4095=ORIENTED_EDGE('',*,*,#3197,.F.);
#4096=ORIENTED_EDGE('',*,*,#3226,.T.);
#4097=ORIENTED_EDGE('',*,*,#3218,.T.);
#4098=ORIENTED_EDGE('',*,*,#3134,.F.);
#4099=ORIENTED_EDGE('',*,*,#3227,.F.);
#4100=ORIENTED_EDGE('',*,*,#3217,.F.);
#4101=ORIENTED_EDGE('',*,*,#3228,.T.);
#4102=ORIENTED_EDGE('',*,*,#3182,.F.);
#4103=ORIENTED_EDGE('',*,*,#3133,.F.);
#4104=ORIENTED_EDGE('',*,*,#3205,.F.);
#4105=ORIENTED_EDGE('',*,*,#3229,.F.);
#4106=ORIENTED_EDGE('',*,*,#3144,.T.);
#4107=ORIENTED_EDGE('',*,*,#3209,.T.);
#4108=ORIENTED_EDGE('',*,*,#3227,.T.);
#4109=ORIENTED_EDGE('',*,*,#3183,.F.);
#4110=ORIENTED_EDGE('',*,*,#3228,.F.);
#4111=ORIENTED_EDGE('',*,*,#3213,.F.);
#4112=ORIENTED_EDGE('',*,*,#3140,.T.);
#4113=ORIENTED_EDGE('',*,*,#3230,.T.);
#4114=ORIENTED_EDGE('',*,*,#3206,.T.);
#4115=ORIENTED_EDGE('',*,*,#3231,.T.);
#4116=ORIENTED_EDGE('',*,*,#3232,.F.);
#4117=ORIENTED_EDGE('',*,*,#3145,.F.);
#4118=ORIENTED_EDGE('',*,*,#3229,.T.);
#4119=ORIENTED_EDGE('',*,*,#3233,.F.);
#4120=ORIENTED_EDGE('',*,*,#3230,.F.);
#4121=ORIENTED_EDGE('',*,*,#3139,.T.);
#4122=ORIENTED_EDGE('',*,*,#3234,.T.);
#4123=ORIENTED_EDGE('',*,*,#3235,.T.);
#4124=ORIENTED_EDGE('',*,*,#3234,.F.);
#4125=ORIENTED_EDGE('',*,*,#3146,.F.);
#4126=ORIENTED_EDGE('',*,*,#3232,.T.);
#4127=ORIENTED_EDGE('',*,*,#3236,.T.);
#4128=ORIENTED_EDGE('',*,*,#3207,.F.);
#4129=ORIENTED_EDGE('',*,*,#3233,.T.);
#4130=ORIENTED_EDGE('',*,*,#3237,.F.);
#4131=ORIENTED_EDGE('',*,*,#3204,.T.);
#4132=ORIENTED_EDGE('',*,*,#3238,.T.);
#4133=ORIENTED_EDGE('',*,*,#3239,.F.);
#4134=ORIENTED_EDGE('',*,*,#3231,.F.);
#4135=ORIENTED_EDGE('',*,*,#3176,.T.);
#4136=ORIENTED_EDGE('',*,*,#3237,.T.);
#4137=ORIENTED_EDGE('',*,*,#3235,.F.);
#4138=ORIENTED_EDGE('',*,*,#3239,.T.);
#4139=ORIENTED_EDGE('',*,*,#3131,.F.);
#4140=ORIENTED_EDGE('',*,*,#3200,.T.);
#4141=ORIENTED_EDGE('',*,*,#3177,.T.);
#4142=ORIENTED_EDGE('',*,*,#3238,.F.);
#4143=ORIENTED_EDGE('',*,*,#3185,.F.);
#4144=ORIENTED_EDGE('',*,*,#3236,.F.);
#4145=ORIENTED_EDGE('',*,*,#3175,.F.);
#4146=ORIENTED_EDGE('',*,*,#3203,.T.);
#4147=ORIENTED_EDGE('',*,*,#3225,.F.);
#4148=ORIENTED_EDGE('',*,*,#3240,.F.);
#4149=ORIENTED_EDGE('',*,*,#3241,.F.);
#4150=ORIENTED_EDGE('',*,*,#3170,.F.);
#4151=ORIENTED_EDGE('',*,*,#3199,.T.);
#4152=ORIENTED_EDGE('',*,*,#3147,.T.);
#4153=ORIENTED_EDGE('',*,*,#3191,.T.);
#4154=ORIENTED_EDGE('',*,*,#3173,.T.);
#4155=ORIENTED_EDGE('',*,*,#3242,.T.);
#4156=ORIENTED_EDGE('',*,*,#3243,.T.);
#4157=ORIENTED_EDGE('',*,*,#3223,.T.);
#4158=ORIENTED_EDGE('',*,*,#3195,.T.);
#4159=ORIENTED_EDGE('',*,*,#3158,.F.);
#4160=ORIENTED_EDGE('',*,*,#3201,.T.);
#4161=ORIENTED_EDGE('',*,*,#3241,.T.);
#4162=ORIENTED_EDGE('',*,*,#3244,.T.);
#4163=ORIENTED_EDGE('',*,*,#3245,.F.);
#4164=ORIENTED_EDGE('',*,*,#3244,.F.);
#4165=ORIENTED_EDGE('',*,*,#3240,.T.);
#4166=ORIENTED_EDGE('',*,*,#3245,.T.);
#4167=ORIENTED_EDGE('',*,*,#3246,.F.);
#4168=ORIENTED_EDGE('',*,*,#3242,.F.);
#4169=ORIENTED_EDGE('',*,*,#3243,.F.);
#4170=ORIENTED_EDGE('',*,*,#3247,.T.);
#4171=ORIENTED_EDGE('',*,*,#3248,.T.);
#4172=ORIENTED_EDGE('',*,*,#3247,.F.);
#4173=ORIENTED_EDGE('',*,*,#3248,.F.);
#4174=ORIENTED_EDGE('',*,*,#3168,.F.);
#4175=ORIENTED_EDGE('',*,*,#3164,.F.);
#4176=ORIENTED_EDGE('',*,*,#3165,.F.);
#4177=ORIENTED_EDGE('',*,*,#3249,.T.);
#4178=ORIENTED_EDGE('',*,*,#3246,.T.);
#4179=ORIENTED_EDGE('',*,*,#3249,.F.);
#4180=ORIENTED_EDGE('',*,*,#3250,.T.);
#4181=ORIENTED_EDGE('',*,*,#3163,.F.);
#4182=ORIENTED_EDGE('',*,*,#3250,.F.);
#4183=ORIENTED_EDGE('',*,*,#3251,.T.);
#4184=ORIENTED_EDGE('',*,*,#3171,.T.);
#4185=ORIENTED_EDGE('',*,*,#3224,.T.);
#4186=ORIENTED_EDGE('',*,*,#3172,.T.);
#4187=ORIENTED_EDGE('',*,*,#3251,.F.);
#4188=ORIENTED_EDGE('',*,*,#3161,.T.);
#4189=ORIENTED_EDGE('',*,*,#3179,.T.);
#4190=ORIENTED_EDGE('',*,*,#3202,.F.);
#4191=ORIENTED_EDGE('',*,*,#3160,.F.);
#4192=ORIENTED_EDGE('',*,*,#3194,.T.);
#4193=ORIENTED_EDGE('',*,*,#3129,.F.);
#4194=ORIENTED_EDGE('',*,*,#3192,.F.);
#4195=ORIENTED_EDGE('',*,*,#3149,.T.);
#4196=ORIENTED_EDGE('',*,*,#3198,.T.);
#4197=ORIENTED_EDGE('',*,*,#3156,.T.);
#4198=ORIENTED_EDGE('',*,*,#3252,.T.);
#4199=ORIENTED_EDGE('',*,*,#3138,.T.);
#4200=ORIENTED_EDGE('',*,*,#3252,.F.);
#4201=ORIENTED_EDGE('',*,*,#3155,.T.);
#4202=ORIENTED_EDGE('',*,*,#3253,.T.);
#4203=ORIENTED_EDGE('',*,*,#3137,.T.);
#4204=ORIENTED_EDGE('',*,*,#3253,.F.);
#4205=ORIENTED_EDGE('',*,*,#3154,.T.);
#4206=ORIENTED_EDGE('',*,*,#3254,.T.);
#4207=ORIENTED_EDGE('',*,*,#3136,.T.);
#4208=ORIENTED_EDGE('',*,*,#3254,.F.);
#4209=ORIENTED_EDGE('',*,*,#3153,.F.);
#4210=ORIENTED_EDGE('',*,*,#3255,.T.);
#4211=ORIENTED_EDGE('',*,*,#3189,.F.);
#4212=ORIENTED_EDGE('',*,*,#3255,.F.);
#4213=ORIENTED_EDGE('',*,*,#3152,.F.);
#4214=ORIENTED_EDGE('',*,*,#3256,.T.);
#4215=ORIENTED_EDGE('',*,*,#3188,.F.);
#4216=ORIENTED_EDGE('',*,*,#3256,.F.);
#4217=ORIENTED_EDGE('',*,*,#3151,.F.);
#4218=ORIENTED_EDGE('',*,*,#3257,.T.);
#4219=ORIENTED_EDGE('',*,*,#3187,.F.);
#4220=ORIENTED_EDGE('',*,*,#3257,.F.);
#5627=PLANE('',#6260);
#5628=PLANE('',#6265);
#5629=PLANE('',#6288);
#5630=PLANE('',#6293);
#5631=PLANE('',#6295);
#5632=PLANE('',#6297);
#5633=PLANE('',#6298);
#5634=PLANE('',#6299);
#5635=PLANE('',#6300);
#5636=PLANE('',#6305);
#5637=PLANE('',#6306);
#5638=PLANE('',#6312);
#5639=PLANE('',#6315);
#5640=PLANE('',#6320);
#5641=PLANE('',#6324);
#5642=PLANE('',#6326);
#5643=PLANE('',#6329);
#5644=PLANE('',#6330);
#5645=PLANE('',#6331);
#5781=ADVANCED_FACE('',(#732,#627,#628,#629),#5627,.T.);
#5782=ADVANCED_FACE('',(#733,#630,#631,#632,#633,#634,#635,#636,#637),#5628,
 .T.);
#5783=ADVANCED_FACE('',(#734,#638,#639),#477,.F.);
#5784=ADVANCED_FACE('',(#735),#478,.F.);
#5785=ADVANCED_FACE('',(#736),#479,.T.);
#5786=ADVANCED_FACE('',(#737,#640,#641,#642),#5629,.T.);
#5787=ADVANCED_FACE('',(#738),#5630,.T.);
#5788=ADVANCED_FACE('',(#739),#5631,.T.);
#5789=ADVANCED_FACE('',(#740),#5632,.T.);
#5790=ADVANCED_FACE('',(#741),#5633,.T.);
#5791=ADVANCED_FACE('',(#742),#5634,.T.);
#5792=ADVANCED_FACE('',(#743),#5635,.T.);
#5793=ADVANCED_FACE('',(#744),#480,.F.);
#5794=ADVANCED_FACE('',(#745),#481,.F.);
#5795=ADVANCED_FACE('',(#746),#482,.T.);
#5796=ADVANCED_FACE('',(#747),#279,.T.);
#5797=ADVANCED_FACE('',(#748),#280,.T.);
#5798=ADVANCED_FACE('',(#749),#281,.T.);
#5799=ADVANCED_FACE('',(#750),#282,.F.);
#5800=ADVANCED_FACE('',(#751),#483,.T.);
#5801=ADVANCED_FACE('',(#752),#283,.F.);
#5802=ADVANCED_FACE('',(#753),#5636,.T.);
#5803=ADVANCED_FACE('',(#754),#5637,.T.);
#5804=ADVANCED_FACE('',(#755),#484,.T.);
#5805=ADVANCED_FACE('',(#756),#485,.T.);
#5806=ADVANCED_FACE('',(#757),#486,.F.);
#5807=ADVANCED_FACE('',(#758),#487,.F.);
#5808=ADVANCED_FACE('',(#759),#488,.T.);
#5809=ADVANCED_FACE('',(#760),#284,.F.);
#5810=ADVANCED_FACE('',(#761),#285,.F.);
#5811=ADVANCED_FACE('',(#762),#286,.F.);
#5812=ADVANCED_FACE('',(#763),#287,.T.);
#5813=ADVANCED_FACE('',(#764),#288,.T.);
#5814=ADVANCED_FACE('',(#765),#5638,.F.);
#5815=ADVANCED_FACE('',(#766),#5639,.F.);
#5816=ADVANCED_FACE('',(#767),#489,.T.);
#5817=ADVANCED_FACE('',(#768,#643),#5640,.T.);
#5818=ADVANCED_FACE('',(#769),#490,.T.);
#5819=ADVANCED_FACE('',(#770,#644),#5641,.T.);
#5820=ADVANCED_FACE('',(#771),#491,.F.);
#5821=ADVANCED_FACE('',(#772,#645),#5642,.T.);
#5822=ADVANCED_FACE('',(#773),#492,.T.);
#5823=ADVANCED_FACE('',(#774),#5643,.F.);
#5824=ADVANCED_FACE('',(#775),#5644,.F.);
#5825=ADVANCED_FACE('',(#776),#5645,.T.);
#5826=ADVANCED_FACE('',(#777),#493,.F.);
#5827=ADVANCED_FACE('',(#778),#494,.F.);
#5828=ADVANCED_FACE('',(#779),#495,.F.);
#5829=ADVANCED_FACE('',(#780),#496,.F.);
#5830=ADVANCED_FACE('',(#781),#497,.F.);
#5831=ADVANCED_FACE('',(#782),#498,.F.);
#6134=CLOSED_SHELL('',(#5781,#5782,#5783,#5784,#5785,#5786,#5787,#5788,
#5789,#5790,#5791,#5792,#5793,#5794,#5795,#5796,#5797,#5798,#5799,#5800,
#5801,#5802,#5803,#5804,#5805,#5806,#5807,#5808,#5809,#5810,#5811,#5812,
#5813,#5814,#5815,#5816,#5817,#5818,#5819,#5820,#5821,#5822,#5823,#5824,
#5825,#5826,#5827,#5828,#5829,#5830,#5831));
#6259=AXIS2_PLACEMENT_3D('',#8594,#6909,#6910);
#6260=AXIS2_PLACEMENT_3D('',#8595,#6911,#6912);
#6261=AXIS2_PLACEMENT_3D('',#8608,#6918,#6919);
#6262=AXIS2_PLACEMENT_3D('',#8613,#6922,#6923);
#6263=AXIS2_PLACEMENT_3D('',#8615,#6924,#6925);
#6264=AXIS2_PLACEMENT_3D('',#8617,#6926,#6927);
#6265=AXIS2_PLACEMENT_3D('',#8618,#6928,#6929);
#6266=AXIS2_PLACEMENT_3D('',#8621,#6930,#6931);
#6267=AXIS2_PLACEMENT_3D('',#8623,#6932,#6933);
#6268=AXIS2_PLACEMENT_3D('',#8625,#6934,#6935);
#6269=AXIS2_PLACEMENT_3D('',#8627,#6936,#6937);
#6270=AXIS2_PLACEMENT_3D('',#8629,#6938,#6939);
#6271=AXIS2_PLACEMENT_3D('',#8631,#6940,#6941);
#6272=AXIS2_PLACEMENT_3D('',#8633,#6942,#6943);
#6273=AXIS2_PLACEMENT_3D('',#8634,#6944,#6945);
#6274=AXIS2_PLACEMENT_3D('',#8644,#6950,#6951);
#6275=AXIS2_PLACEMENT_3D('',#8646,#6952,#6953);
#6276=AXIS2_PLACEMENT_3D('',#8648,#6954,#6955);
#6277=AXIS2_PLACEMENT_3D('',#8650,#6956,#6957);
#6278=AXIS2_PLACEMENT_3D('',#8652,#6958,#6959);
#6279=AXIS2_PLACEMENT_3D('',#8654,#6960,#6961);
#6280=AXIS2_PLACEMENT_3D('',#8663,#6966,#6967);
#6281=AXIS2_PLACEMENT_3D('',#8665,#6968,#6969);
#6282=AXIS2_PLACEMENT_3D('',#8668,#6971,#6972);
#6283=AXIS2_PLACEMENT_3D('',#8825,#6973,#6974);
#6284=AXIS2_PLACEMENT_3D('',#8827,#6975,#6976);
#6285=AXIS2_PLACEMENT_3D('',#8829,#6978,#6979);
#6286=AXIS2_PLACEMENT_3D('',#8874,#6982,#6983);
#6287=AXIS2_PLACEMENT_3D('',#8905,#6986,#6987);
#6288=AXIS2_PLACEMENT_3D('',#8906,#6988,#6989);
#6289=AXIS2_PLACEMENT_3D('',#8917,#6994,#6995);
#6290=AXIS2_PLACEMENT_3D('',#8924,#6999,#7000);
#6291=AXIS2_PLACEMENT_3D('',#8926,#7001,#7002);
#6292=AXIS2_PLACEMENT_3D('',#8928,#7003,#7004);
#6293=AXIS2_PLACEMENT_3D('',#8929,#7005,#7006);
#6294=AXIS2_PLACEMENT_3D('',#8932,#7007,#7008);
#6295=AXIS2_PLACEMENT_3D('',#9119,#7011,#7012);
#6296=AXIS2_PLACEMENT_3D('',#9124,#7015,#7016);
#6297=AXIS2_PLACEMENT_3D('',#9306,#7017,#7018);
#6298=AXIS2_PLACEMENT_3D('',#9313,#7021,#7022);
#6299=AXIS2_PLACEMENT_3D('',#9320,#7025,#7026);
#6300=AXIS2_PLACEMENT_3D('',#9327,#7028,#7029);
#6301=AXIS2_PLACEMENT_3D('',#9336,#7031,#7032);
#6302=AXIS2_PLACEMENT_3D('',#9387,#7035,#7036);
#6303=AXIS2_PLACEMENT_3D('',#9438,#7039,#7040);
#6304=AXIS2_PLACEMENT_3D('',#9732,#7044,#7045);
#6305=AXIS2_PLACEMENT_3D('',#9778,#7049,#7050);
#6306=AXIS2_PLACEMENT_3D('',#9780,#7052,#7053);
#6307=AXIS2_PLACEMENT_3D('',#9782,#7055,#7056);
#6308=AXIS2_PLACEMENT_3D('',#9784,#7058,#7059);
#6309=AXIS2_PLACEMENT_3D('',#9786,#7061,#7062);
#6310=AXIS2_PLACEMENT_3D('',#9835,#7064,#7065);
#6311=AXIS2_PLACEMENT_3D('',#9884,#7067,#7068);
#6312=AXIS2_PLACEMENT_3D('',#10148,#7071,#7072);
#6313=AXIS2_PLACEMENT_3D('',#10150,#7073,#7074);
#6314=AXIS2_PLACEMENT_3D('',#10151,#7075,#7076);
#6315=AXIS2_PLACEMENT_3D('',#10152,#7077,#7078);
#6316=AXIS2_PLACEMENT_3D('',#10154,#7079,#7080);
#6317=AXIS2_PLACEMENT_3D('',#10155,#7081,#7082);
#6318=AXIS2_PLACEMENT_3D('',#10156,#7083,#7084);
#6319=AXIS2_PLACEMENT_3D('',#10159,#7086,#7087);
#6320=AXIS2_PLACEMENT_3D('',#10160,#7088,#7089);
#6321=AXIS2_PLACEMENT_3D('',#10162,#7090,#7091);
#6322=AXIS2_PLACEMENT_3D('',#10163,#7092,#7093);
#6323=AXIS2_PLACEMENT_3D('',#10166,#7095,#7096);
#6324=AXIS2_PLACEMENT_3D('',#10167,#7097,#7098);
#6325=AXIS2_PLACEMENT_3D('',#10168,#7099,#7100);
#6326=AXIS2_PLACEMENT_3D('',#10170,#7102,#7103);
#6327=AXIS2_PLACEMENT_3D('',#10172,#7104,#7105);
#6328=AXIS2_PLACEMENT_3D('',#10173,#7106,#7107);
#6329=AXIS2_PLACEMENT_3D('',#10175,#7109,#7110);
#6330=AXIS2_PLACEMENT_3D('',#10176,#7111,#7112);
#6331=AXIS2_PLACEMENT_3D('',#10177,#7113,#7114);
#6332=AXIS2_PLACEMENT_3D('',#10178,#7115,#7116);
#6333=AXIS2_PLACEMENT_3D('',#10180,#7118,#7119);
#6334=AXIS2_PLACEMENT_3D('',#10182,#7121,#7122);
#6335=AXIS2_PLACEMENT_3D('',#10184,#7124,#7125);
#6336=AXIS2_PLACEMENT_3D('',#10186,#7127,#7128);
#6337=AXIS2_PLACEMENT_3D('',#10188,#7130,#7131);
#6909=DIRECTION('axis',(0.,0.,1.));
#6910=DIRECTION('refdir',(1.,0.,0.));
#6911=DIRECTION('center_axis',(0.,1.,0.));
#6912=DIRECTION('ref_axis',(0.,0.,1.));
#6913=DIRECTION('',(1.,0.,-1.4799935157375E-16));
#6914=DIRECTION('',(0.,0.,-1.));
#6915=DIRECTION('',(1.,0.,-1.47999351573749E-16));
#6916=DIRECTION('',(0.,3.88578058618804E-16,-1.));
#6917=DIRECTION('',(-1.,0.,0.));
#6918=DIRECTION('center_axis',(0.,1.,0.));
#6919=DIRECTION('ref_axis',(0.,0.,1.));
#6920=DIRECTION('',(1.,0.,-4.40139925476306E-16));
#6921=DIRECTION('',(0.,0.,1.));
#6922=DIRECTION('center_axis',(0.,1.,0.));
#6923=DIRECTION('ref_axis',(0.,0.,-1.));
#6924=DIRECTION('center_axis',(0.,1.,0.));
#6925=DIRECTION('ref_axis',(0.,0.,1.));
#6926=DIRECTION('center_axis',(0.,1.,0.));
#6927=DIRECTION('ref_axis',(0.,0.,1.));
#6928=DIRECTION('center_axis',(0.,-1.,0.));
#6929=DIRECTION('ref_axis',(0.,0.,-1.));
#6930=DIRECTION('center_axis',(-7.86509422263479E-32,-1.,-4.2478565844662E-16));
#6931=DIRECTION('ref_axis',(-3.70308840058128E-16,4.24785658446619E-16,
-1.));
#6932=DIRECTION('center_axis',(0.,1.,0.));
#6933=DIRECTION('ref_axis',(0.,0.,-1.));
#6934=DIRECTION('center_axis',(0.,1.,0.));
#6935=DIRECTION('ref_axis',(0.,0.,1.));
#6936=DIRECTION('center_axis',(0.,1.,0.));
#6937=DIRECTION('ref_axis',(0.,0.,1.));
#6938=DIRECTION('center_axis',(0.,-1.,0.));
#6939=DIRECTION('ref_axis',(0.,0.,-1.));
#6940=DIRECTION('center_axis',(0.,1.,0.));
#6941=DIRECTION('ref_axis',(0.,0.,1.));
#6942=DIRECTION('center_axis',(7.86509422263479E-32,1.,4.2478565844662E-16));
#6943=DIRECTION('ref_axis',(3.70308840058128E-16,-4.2478565844662E-16,1.));
#6944=DIRECTION('center_axis',(-7.86509422263479E-32,-1.,-4.2478565844662E-16));
#6945=DIRECTION('ref_axis',(-3.70308840058128E-16,4.24785658446619E-16,
-1.));
#6946=DIRECTION('',(-2.10042193848003E-16,0.,1.));
#6947=DIRECTION('',(1.,0.,3.88971843979164E-16));
#6948=DIRECTION('',(0.,0.,-1.));
#6949=DIRECTION('',(-1.,0.,0.));
#6950=DIRECTION('center_axis',(0.,-1.,0.));
#6951=DIRECTION('ref_axis',(0.,0.,-1.));
#6952=DIRECTION('center_axis',(0.,-1.,0.));
#6953=DIRECTION('ref_axis',(0.,0.,-1.));
#6954=DIRECTION('center_axis',(0.,-1.,0.));
#6955=DIRECTION('ref_axis',(0.,0.,-1.));
#6956=DIRECTION('center_axis',(0.,-1.,0.));
#6957=DIRECTION('ref_axis',(0.,0.,-1.));
#6958=DIRECTION('center_axis',(0.,-1.,0.));
#6959=DIRECTION('ref_axis',(0.,0.,-1.));
#6960=DIRECTION('center_axis',(0.,-1.,0.));
#6961=DIRECTION('ref_axis',(0.,0.,-1.));
#6962=DIRECTION('',(-1.,0.,3.88971843979164E-16));
#6963=DIRECTION('',(2.10042193848003E-16,0.,1.));
#6964=DIRECTION('',(1.,0.,0.));
#6965=DIRECTION('',(0.,0.,-1.));
#6966=DIRECTION('center_axis',(0.,1.,0.));
#6967=DIRECTION('ref_axis',(0.,0.,1.));
#6968=DIRECTION('center_axis',(0.,-1.,0.));
#6969=DIRECTION('ref_axis',(0.,0.,-1.));
#6970=DIRECTION('',(0.,1.,0.));
#6971=DIRECTION('center_axis',(0.,1.,0.));
#6972=DIRECTION('ref_axis',(0.,0.,1.));
#6973=DIRECTION('center_axis',(-1.,1.4811191380744E-16,1.85154420029064E-16));
#6974=DIRECTION('ref_axis',(1.85154420029064E-16,0.,1.));
#6975=DIRECTION('center_axis',(1.,1.4811191380744E-16,1.85154420029064E-16));
#6976=DIRECTION('ref_axis',(1.85154420029064E-16,0.,-1.));
#6977=DIRECTION('',(-1.,1.4811191380744E-16,1.85154420029064E-16));
#6978=DIRECTION('center_axis',(2.37862219570569E-17,0.,1.));
#6979=DIRECTION('ref_axis',(1.,0.,-2.37862219570569E-17));
#6980=DIRECTION('',(1.20024110770287E-16,-4.80096443081149E-16,1.));
#6981=DIRECTION('',(2.40048221540575E-16,-4.80096443081149E-16,1.));
#6982=DIRECTION('center_axis',(-3.46522618101071E-16,4.2478565844662E-16,
-1.));
#6983=DIRECTION('ref_axis',(-1.,-6.8546896270362E-32,3.46522618101071E-16));
#6984=DIRECTION('',(0.,0.,-1.));
#6985=DIRECTION('',(0.,0.,-1.));
#6986=DIRECTION('center_axis',(-3.46522618101071E-16,4.2478565844662E-16,
-1.));
#6987=DIRECTION('ref_axis',(-1.,-6.8546896270362E-32,3.46522618101071E-16));
#6988=DIRECTION('center_axis',(0.,1.,0.));
#6989=DIRECTION('ref_axis',(0.,0.,1.));
#6990=DIRECTION('',(0.,0.,-1.));
#6991=DIRECTION('',(1.,0.,-1.47999270653708E-16));
#6992=DIRECTION('',(0.,0.,1.));
#6993=DIRECTION('',(1.,0.,0.));
#6994=DIRECTION('center_axis',(0.,1.,0.));
#6995=DIRECTION('ref_axis',(0.,0.,-1.));
#6996=DIRECTION('',(-1.,0.,4.40139925486788E-16));
#6997=DIRECTION('',(0.,3.88578058618805E-16,-1.));
#6998=DIRECTION('',(1.,0.,-2.95998541307373E-16));
#6999=DIRECTION('center_axis',(0.,-1.,0.));
#7000=DIRECTION('ref_axis',(0.,0.,-1.));
#7001=DIRECTION('center_axis',(0.,-1.,0.));
#7002=DIRECTION('ref_axis',(0.,0.,1.));
#7003=DIRECTION('center_axis',(0.,-1.,0.));
#7004=DIRECTION('ref_axis',(0.,0.,1.));
#7005=DIRECTION('center_axis',(-1.85154420029064E-16,2.1239282922331E-16,
-1.));
#7006=DIRECTION('ref_axis',(-1.,0.,1.85154420029064E-16));
#7007=DIRECTION('center_axis',(-2.37862219570569E-17,0.,-1.));
#7008=DIRECTION('ref_axis',(-1.,0.,2.37862219570569E-17));
#7009=DIRECTION('',(2.30359800135544E-16,1.,1.72769850101658E-16));
#7010=DIRECTION('',(0.,1.,0.));
#7011=DIRECTION('center_axis',(-1.85154420029064E-16,2.1239282922331E-16,
-1.));
#7012=DIRECTION('ref_axis',(-1.,0.,1.85154420029064E-16));
#7013=DIRECTION('',(0.,1.,0.));
#7014=DIRECTION('',(-5.7589950033886E-17,-1.,-2.30359800135544E-16));
#7015=DIRECTION('center_axis',(-2.37862219570569E-17,0.,-1.));
#7016=DIRECTION('ref_axis',(-1.,0.,2.37862219570569E-17));
#7017=DIRECTION('center_axis',(1.85154420029064E-16,-2.1239282922331E-16,
1.));
#7018=DIRECTION('ref_axis',(1.,0.,-1.85154420029064E-16));
#7019=DIRECTION('',(0.,1.,0.));
#7020=DIRECTION('',(-2.30359800135544E-16,-1.,-1.15179900067772E-16));
#7021=DIRECTION('center_axis',(1.85154420029064E-16,-2.1239282922331E-16,
1.));
#7022=DIRECTION('ref_axis',(1.,0.,-1.85154420029064E-16));
#7023=DIRECTION('',(2.8794975016943E-17,1.,2.30359800135544E-16));
#7024=DIRECTION('',(0.,1.,0.));
#7025=DIRECTION('center_axis',(-6.3741727053016E-17,0.,-1.));
#7026=DIRECTION('ref_axis',(-1.,0.,6.3741727053016E-17));
#7027=DIRECTION('',(0.,1.,0.));
#7028=DIRECTION('center_axis',(-6.3741727053016E-17,0.,-1.));
#7029=DIRECTION('ref_axis',(-1.,0.,6.3741727053016E-17));
#7030=DIRECTION('',(0.,1.,0.));
#7031=DIRECTION('center_axis',(0.,1.,0.));
#7032=DIRECTION('ref_axis',(0.,0.,1.));
#7033=DIRECTION('',(0.,1.,0.));
#7034=DIRECTION('',(0.,1.,0.));
#7035=DIRECTION('center_axis',(0.,1.,0.));
#7036=DIRECTION('ref_axis',(0.,0.,1.));
#7037=DIRECTION('',(0.,1.,0.));
#7038=DIRECTION('',(0.,1.,0.));
#7039=DIRECTION('center_axis',(0.,1.,0.));
#7040=DIRECTION('ref_axis',(0.,0.,1.));
#7041=DIRECTION('',(-0.00148924434041068,-0.517944475025485,0.855412942935673));
#7042=DIRECTION('',(-0.0014892443404113,0.517944475025485,-0.855412942935673));
#7043=DIRECTION('',(0.,0.,1.));
#7044=DIRECTION('center_axis',(2.37862219570569E-17,0.,1.));
#7045=DIRECTION('ref_axis',(1.,0.,-2.37862219570569E-17));
#7046=DIRECTION('',(1.80036166155431E-16,0.,1.));
#7047=DIRECTION('',(2.40048221540574E-16,0.,1.));
#7048=DIRECTION('',(0.,0.,1.));
#7049=DIRECTION('center_axis',(6.3741727053016E-17,0.,1.));
#7050=DIRECTION('ref_axis',(1.,0.,-6.3741727053016E-17));
#7051=DIRECTION('',(0.,1.,0.));
#7052=DIRECTION('center_axis',(6.3741727053016E-17,0.,1.));
#7053=DIRECTION('ref_axis',(1.,0.,-6.3741727053016E-17));
#7054=DIRECTION('',(0.,1.,0.));
#7055=DIRECTION('center_axis',(0.,1.,0.));
#7056=DIRECTION('ref_axis',(0.,0.,1.));
#7057=DIRECTION('',(0.,1.,0.));
#7058=DIRECTION('center_axis',(0.,1.,0.));
#7059=DIRECTION('ref_axis',(0.,0.,1.));
#7060=DIRECTION('',(0.,1.,0.));
#7061=DIRECTION('center_axis',(7.86509422263479E-32,1.,4.2478565844662E-16));
#7062=DIRECTION('ref_axis',(-3.70308840058128E-16,4.2478565844662E-16,-1.));
#7063=DIRECTION('',(0.,1.,0.));
#7064=DIRECTION('center_axis',(7.86509422263479E-32,1.,4.2478565844662E-16));
#7065=DIRECTION('ref_axis',(-3.70308840058128E-16,4.24785658446619E-16,
-1.));
#7066=DIRECTION('',(0.,1.,0.));
#7067=DIRECTION('center_axis',(7.86509422263479E-32,1.,4.2478565844662E-16));
#7068=DIRECTION('ref_axis',(-3.70308840058128E-16,4.24785658446619E-16,
-1.));
#7069=DIRECTION('',(-0.00148924434041153,-0.517944475025485,-0.855412942935673));
#7070=DIRECTION('',(-0.00148924434041087,0.517944475025484,0.855412942935674));
#7071=DIRECTION('center_axis',(1.,-2.06784640888072E-16,-1.85154420029064E-16));
#7072=DIRECTION('ref_axis',(-1.85154420029064E-16,0.,-1.));
#7073=DIRECTION('center_axis',(-1.,1.4811191380744E-16,1.85154420029064E-16));
#7074=DIRECTION('ref_axis',(1.85154420029064E-16,0.,1.));
#7075=DIRECTION('center_axis',(-1.,1.4811191380744E-16,1.85154420029064E-16));
#7076=DIRECTION('ref_axis',(1.85154420029064E-16,0.,1.));
#7077=DIRECTION('center_axis',(-1.,5.16961602220179E-17,1.85154420029064E-16));
#7078=DIRECTION('ref_axis',(1.85154420029064E-16,0.,1.));
#7079=DIRECTION('center_axis',(-1.,-1.4811191380744E-16,-1.85154420029064E-16));
#7080=DIRECTION('ref_axis',(-1.85154420029064E-16,0.,1.));
#7081=DIRECTION('center_axis',(-1.,-1.4811191380744E-16,-1.85154420029064E-16));
#7082=DIRECTION('ref_axis',(-1.85154420029064E-16,0.,1.));
#7083=DIRECTION('center_axis',(1.,-1.4811191380744E-16,-1.85154420029064E-16));
#7084=DIRECTION('ref_axis',(-1.85154420029064E-16,0.,-1.));
#7085=DIRECTION('',(-1.,1.4811191380744E-16,1.85154420029064E-16));
#7086=DIRECTION('center_axis',(-1.,1.4811191380744E-16,1.85154420029064E-16));
#7087=DIRECTION('ref_axis',(1.85154420029064E-16,0.,1.));
#7088=DIRECTION('center_axis',(-1.,1.4811191380744E-16,1.85154420029064E-16));
#7089=DIRECTION('ref_axis',(1.85154420029064E-16,0.,1.));
#7090=DIRECTION('center_axis',(-1.,1.4811191380744E-16,1.85154420029064E-16));
#7091=DIRECTION('ref_axis',(1.85154420029064E-16,0.,1.));
#7092=DIRECTION('center_axis',(-1.,-1.4811191380744E-16,-1.85154420029064E-16));
#7093=DIRECTION('ref_axis',(-1.85154420029064E-16,0.,1.));
#7094=DIRECTION('',(1.,1.4811191380744E-16,1.85154420029064E-16));
#7095=DIRECTION('center_axis',(-1.,-1.4811191380744E-16,-1.85154420029064E-16));
#7096=DIRECTION('ref_axis',(-1.85154420029064E-16,0.,1.));
#7097=DIRECTION('center_axis',(1.,1.4811191380744E-16,1.85154420029064E-16));
#7098=DIRECTION('ref_axis',(1.85154420029064E-16,0.,-1.));
#7099=DIRECTION('center_axis',(-1.,1.4811191380744E-16,1.85154420029064E-16));
#7100=DIRECTION('ref_axis',(1.85154420029064E-16,0.,1.));
#7101=DIRECTION('',(-1.,1.4811191380744E-16,1.85154420029064E-16));
#7102=DIRECTION('center_axis',(0.,1.,0.));
#7103=DIRECTION('ref_axis',(0.,0.,1.));
#7104=DIRECTION('center_axis',(0.,1.,0.));
#7105=DIRECTION('ref_axis',(0.,0.,1.));
#7106=DIRECTION('center_axis',(0.,1.,0.));
#7107=DIRECTION('ref_axis',(0.,0.,1.));
#7108=DIRECTION('',(0.,-1.,0.));
#7109=DIRECTION('center_axis',(0.,-1.,0.));
#7110=DIRECTION('ref_axis',(0.,0.,-1.));
#7111=DIRECTION('center_axis',(1.,0.,0.));
#7112=DIRECTION('ref_axis',(0.,0.,-1.));
#7113=DIRECTION('center_axis',(1.,0.,0.));
#7114=DIRECTION('ref_axis',(0.,0.,-1.));
#7115=DIRECTION('center_axis',(0.,1.,0.));
#7116=DIRECTION('ref_axis',(0.,0.,1.));
#7117=DIRECTION('',(0.,1.,0.));
#7118=DIRECTION('center_axis',(0.,1.,0.));
#7119=DIRECTION('ref_axis',(0.,0.,1.));
#7120=DIRECTION('',(0.,1.,0.));
#7121=DIRECTION('center_axis',(0.,1.,0.));
#7122=DIRECTION('ref_axis',(0.,0.,1.));
#7123=DIRECTION('',(0.,1.,0.));
#7124=DIRECTION('center_axis',(0.,1.,0.));
#7125=DIRECTION('ref_axis',(0.,0.,1.));
#7126=DIRECTION('',(0.,1.,0.));
#7127=DIRECTION('center_axis',(0.,1.,0.));
#7128=DIRECTION('ref_axis',(0.,0.,1.));
#7129=DIRECTION('',(0.,1.,0.));
#7130=DIRECTION('center_axis',(0.,1.,0.));
#7131=DIRECTION('ref_axis',(0.,0.,1.));
#7132=DIRECTION('',(0.,1.,0.));
#8594=CARTESIAN_POINT('',(0.,0.,0.));
#8595=CARTESIAN_POINT('Origin',(-99.7519848385422,5.,-11.9999999999999));
#8596=CARTESIAN_POINT('',(-125.680065601265,5.,25.0000000000001));
#8597=CARTESIAN_POINT('',(-65.6680057154831,5.,25.0000000000001));
#8598=CARTESIAN_POINT('',(-125.680324030103,5.,25.0000000000001));
#8599=CARTESIAN_POINT('',(-65.6680057154831,5.,-48.9999999999999));
#8600=CARTESIAN_POINT('',(-65.6680057154831,5.,25.0000000000001));
#8601=CARTESIAN_POINT('',(-125.680065601265,5.00000000000001,-48.9999999999999));
#8602=CARTESIAN_POINT('',(-125.680324030103,5.,-48.9999999999999));
#8603=CARTESIAN_POINT('',(-125.68006560189,4.99999999980206,-58.9999999999999));
#8604=CARTESIAN_POINT('',(-125.680065601265,5.,-48.9999999999999));
#8605=CARTESIAN_POINT('',(-145.859521458148,5.,-58.9999999999999));
#8606=CARTESIAN_POINT('',(-125.680065601745,5.,-58.9999999999999));
#8607=CARTESIAN_POINT('',(-145.859521458148,5.,35.0000000000001));
#8608=CARTESIAN_POINT('Origin',(-99.7519848385422,5.,-11.9999999999999));
#8609=CARTESIAN_POINT('',(-125.68006560126,5.00000000000148,35.0000000000001));
#8610=CARTESIAN_POINT('',(-145.859521458148,5.,35.0000000000001));
#8611=CARTESIAN_POINT('',(-125.680065601264,5.,25.0000000000001));
#8612=CARTESIAN_POINT('',(-88.9375988864104,5.,-15.9999999999999));
#8613=CARTESIAN_POINT('Origin',(-88.9375988864104,5.,-11.9999999999999));
#8614=CARTESIAN_POINT('',(-115.629992744845,5.,-27.9631510575948));
#8615=CARTESIAN_POINT('Origin',(-115.629992744845,5.,-11.9999999999999));
#8616=CARTESIAN_POINT('',(-142.322386603279,5.,-15.9999999999999));
#8617=CARTESIAN_POINT('Origin',(-142.322386603279,5.,-11.9999999999999));
#8618=CARTESIAN_POINT('Origin',(-145.859521458148,-5.,144.542028553823));
#8619=CARTESIAN_POINT('',(145.859521458148,-4.99999999999998,-59.));
#8620=CARTESIAN_POINT('',(36.8276756314269,-4.99999999999994,-157.982075177761));
#8621=CARTESIAN_POINT('Origin',(145.859521458148,-4.99999999999993,-168.542028553823));
#8622=CARTESIAN_POINT('',(145.859521458148,-5.,35.0000000000001));
#8623=CARTESIAN_POINT('Origin',(99.7519848385422,-5.,-11.9999999999999));
#8624=CARTESIAN_POINT('',(36.827675631427,-5.,133.982075177761));
#8625=CARTESIAN_POINT('Origin',(145.859521458148,-5.,144.542028553823));
#8626=CARTESIAN_POINT('',(-36.8276756314269,-5.,133.982075177761));
#8627=CARTESIAN_POINT('Origin',(0.,-5.,130.415240784856));
#8628=CARTESIAN_POINT('',(-145.859521458148,-5.,35.0000000000001));
#8629=CARTESIAN_POINT('Origin',(-145.859521458148,-5.,144.542028553823));
#8630=CARTESIAN_POINT('',(-145.859521458148,-4.99999999999998,-58.9999999999999));
#8631=CARTESIAN_POINT('Origin',(-99.7519848385422,-5.,-11.9999999999999));
#8632=CARTESIAN_POINT('',(-36.827675631427,-4.99999999999994,-157.982075177761));
#8633=CARTESIAN_POINT('Origin',(-145.859521458148,-4.99999999999993,-168.542028553823));
#8634=CARTESIAN_POINT('Origin',(-5.2737622621639E-14,-4.99999999999994,
-154.415240784856));
#8635=CARTESIAN_POINT('',(-20.,-5.,-48.9999999999999));
#8636=CARTESIAN_POINT('',(-20.,-5.,25.0000000000001));
#8637=CARTESIAN_POINT('',(-20.,-5.,-48.9999999999999));
#8638=CARTESIAN_POINT('',(-65.6680057154831,-5.,-48.9999999999999));
#8639=CARTESIAN_POINT('',(-65.6680057154831,-5.,-48.9999999999999));
#8640=CARTESIAN_POINT('',(-65.6680057154831,-5.,25.0000000000001));
#8641=CARTESIAN_POINT('',(-65.6680057154831,-5.,25.0000000000001));
#8642=CARTESIAN_POINT('',(-20.,-5.,25.0000000000001));
#8643=CARTESIAN_POINT('',(88.9375988864104,-5.,-15.9999999999999));
#8644=CARTESIAN_POINT('Origin',(88.9375988864104,-5.,-11.9999999999999));
#8645=CARTESIAN_POINT('',(115.629992744845,-5.,-27.9631510575948));
#8646=CARTESIAN_POINT('Origin',(115.629992744845,-5.,-11.9999999999999));
#8647=CARTESIAN_POINT('',(142.322386603279,-5.,-15.9999999999999));
#8648=CARTESIAN_POINT('Origin',(142.322386603279,-5.,-11.9999999999999));
#8649=CARTESIAN_POINT('',(-88.9375988864104,-5.,-15.9999999999999));
#8650=CARTESIAN_POINT('Origin',(-88.9375988864104,-5.,-11.9999999999999));
#8651=CARTESIAN_POINT('',(-115.629992744845,-5.,-27.9631510575948));
#8652=CARTESIAN_POINT('Origin',(-115.629992744845,-5.,-11.9999999999999));
#8653=CARTESIAN_POINT('',(-142.322386603279,-5.,-15.9999999999999));
#8654=CARTESIAN_POINT('Origin',(-142.322386603279,-5.,-11.9999999999999));
#8655=CARTESIAN_POINT('',(65.6680057154831,-5.,-48.9999999999999));
#8656=CARTESIAN_POINT('',(20.,-5.,-48.9999999999999));
#8657=CARTESIAN_POINT('',(65.6680057154831,-5.,-48.9999999999999));
#8658=CARTESIAN_POINT('',(20.,-5.,25.0000000000001));
#8659=CARTESIAN_POINT('',(20.,-5.,-48.9999999999999));
#8660=CARTESIAN_POINT('',(65.6680057154831,-5.,25.0000000000001));
#8661=CARTESIAN_POINT('',(20.,-5.,25.0000000000001));
#8662=CARTESIAN_POINT('',(65.6680057154831,-5.,25.0000000000001));
#8663=CARTESIAN_POINT('Origin',(0.,-5.00102500000001,-11.9999999999999));
#8664=CARTESIAN_POINT('',(0.,29.,-25.9999999999999));
#8665=CARTESIAN_POINT('Origin',(0.,29.,-11.9999999999999));
#8666=CARTESIAN_POINT('',(-1.71450551880629E-15,89.,-25.9999999999999));
#8667=CARTESIAN_POINT('',(-1.71450551880629E-15,-5.00102500000001,-25.9999999999999));
#8668=CARTESIAN_POINT('Origin',(0.,89.,-11.9999999999999));
#8669=CARTESIAN_POINT('',(-1.6909481438847,54.6122755947453,1.89750676829103));
#8670=CARTESIAN_POINT('',(-1.69094814388458,54.6122755947453,-25.8975067682909));
#8671=CARTESIAN_POINT('Ctrl Pts',(-1.69094814388471,54.6122755947453,1.89750676829103));
#8672=CARTESIAN_POINT('Ctrl Pts',(-1.69094814388471,54.9213889364491,1.89750676829103));
#8673=CARTESIAN_POINT('Ctrl Pts',(-1.76916191043536,55.1731377228307,1.88812065613091));
#8674=CARTESIAN_POINT('Ctrl Pts',(-1.9656264409252,55.6361599846496,1.86167854986234));
#8675=CARTESIAN_POINT('Ctrl Pts',(-2.08733509638717,55.8459330182592,1.84417693298648));
#8676=CARTESIAN_POINT('Ctrl Pts',(-2.48603840542449,56.4613583117431,1.78012768145208));
#8677=CARTESIAN_POINT('Ctrl Pts',(-2.79295687688375,56.8454209830934,1.72280566002277));
#8678=CARTESIAN_POINT('Ctrl Pts',(-3.78895528995958,58.0297922078367,1.49473345638479));
#8679=CARTESIAN_POINT('Ctrl Pts',(-4.53827705470844,58.8319051311986,1.27093230580055));
#8680=CARTESIAN_POINT('Ctrl Pts',(-6.10105549036539,60.4801717461623,0.628963504710961));
#8681=CARTESIAN_POINT('Ctrl Pts',(-6.91295780738778,61.3175968721307,0.21097588427962));
#8682=CARTESIAN_POINT('Ctrl Pts',(-8.49452237285656,62.9386948354568,-0.831293369425304));
#8683=CARTESIAN_POINT('Ctrl Pts',(-9.26451807446147,63.7219839395944,-1.45566578996009));
#8684=CARTESIAN_POINT('Ctrl Pts',(-11.0655427499361,65.5494769648951,-3.28315881526074));
#8685=CARTESIAN_POINT('Ctrl Pts',(-12.116208359012,66.610305038754,-4.74556937837982));
#8686=CARTESIAN_POINT('Ctrl Pts',(-13.2182983629377,67.7220613929565,-7.29533046872904));
#8687=CARTESIAN_POINT('Ctrl Pts',(-13.5094758463079,68.0155297755796,-8.20393179374744));
#8688=CARTESIAN_POINT('Ctrl Pts',(-13.90040638973,68.4094703383725,-10.0778205894963));
#8689=CARTESIAN_POINT('Ctrl Pts',(-14.,68.5097823630363,-11.043174986104));
#8690=CARTESIAN_POINT('Ctrl Pts',(-14.,68.5097823630363,-12.9568250138958));
#8691=CARTESIAN_POINT('Ctrl Pts',(-13.90040638973,68.4094703383725,-13.9221794105036));
#8692=CARTESIAN_POINT('Ctrl Pts',(-13.5094758463079,68.0155297755796,-15.7960682062524));
#8693=CARTESIAN_POINT('Ctrl Pts',(-13.2182983629377,67.7220613929565,-16.7046695312708));
#8694=CARTESIAN_POINT('Ctrl Pts',(-12.116208359012,66.610305038754,-19.25443062162));
#8695=CARTESIAN_POINT('Ctrl Pts',(-11.0655427499361,65.5494769648951,-20.7168411847391));
#8696=CARTESIAN_POINT('Ctrl Pts',(-9.26451807446147,63.7219839395945,-22.5443342100398));
#8697=CARTESIAN_POINT('Ctrl Pts',(-8.49452237285657,62.9386948354569,-23.1687066305745));
#8698=CARTESIAN_POINT('Ctrl Pts',(-6.91295780738777,61.3175968721307,-24.2109758842795));
#8699=CARTESIAN_POINT('Ctrl Pts',(-6.10105549036536,60.4801717461623,-24.6289635047108));
#8700=CARTESIAN_POINT('Ctrl Pts',(-4.53827705470839,58.8319051311986,-25.2709323058004));
#8701=CARTESIAN_POINT('Ctrl Pts',(-3.78895528995955,58.0297922078367,-25.4947334563846));
#8702=CARTESIAN_POINT('Ctrl Pts',(-2.7929568768837,56.8454209830934,-25.7228056600226));
#8703=CARTESIAN_POINT('Ctrl Pts',(-2.48603840542445,56.4613583117431,-25.7801276814519));
#8704=CARTESIAN_POINT('Ctrl Pts',(-2.0873350963871,55.8459330182592,-25.8441769329863));
#8705=CARTESIAN_POINT('Ctrl Pts',(-1.9656264409251,55.6361599846497,-25.8616785498622));
#8706=CARTESIAN_POINT('Ctrl Pts',(-1.76916191043525,55.1731377228307,-25.8881206561308));
#8707=CARTESIAN_POINT('Ctrl Pts',(-1.69094814388459,54.9213889364491,-25.8975067682909));
#8708=CARTESIAN_POINT('Ctrl Pts',(-1.69094814388459,54.6122755947453,-25.8975067682909));
#8709=CARTESIAN_POINT('Ctrl Pts',(-1.69094814388459,54.6122755947453,-25.8975067682909));
#8710=CARTESIAN_POINT('Ctrl Pts',(-1.69094814388459,54.3031622530416,-25.8975067682909));
#8711=CARTESIAN_POINT('Ctrl Pts',(-1.76916191043526,54.05141346666,-25.8881206561308));
#8712=CARTESIAN_POINT('Ctrl Pts',(-1.96562644092511,53.588391204841,-25.8616785498622));
#8713=CARTESIAN_POINT('Ctrl Pts',(-2.08733509638708,53.3786181712314,-25.8441769329863));
#8714=CARTESIAN_POINT('Ctrl Pts',(-2.48603840542441,52.7631928777475,-25.7801276814519));
#8715=CARTESIAN_POINT('Ctrl Pts',(-2.79295687688368,52.3791302063973,-25.7228056600226));
#8716=CARTESIAN_POINT('Ctrl Pts',(-3.78895528995951,51.194758981654,-25.4947334563847));
#8717=CARTESIAN_POINT('Ctrl Pts',(-4.53827705470836,50.3926460582921,-25.2709323058004));
#8718=CARTESIAN_POINT('Ctrl Pts',(-6.10105549036533,48.7443794433284,-24.6289635047108));
#8719=CARTESIAN_POINT('Ctrl Pts',(-6.91295780738773,47.90695431736,-24.2109758842795));
#8720=CARTESIAN_POINT('Ctrl Pts',(-8.49452237285654,46.2858563540338,-23.1687066305746));
#8721=CARTESIAN_POINT('Ctrl Pts',(-9.26451807446145,45.5025672498962,-22.5443342100398));
#8722=CARTESIAN_POINT('Ctrl Pts',(-11.0655427499361,43.6750742245956,-20.7168411847391));
#8723=CARTESIAN_POINT('Ctrl Pts',(-12.116208359012,42.6142461507366,-19.25443062162));
#8724=CARTESIAN_POINT('Ctrl Pts',(-13.2182983629377,41.5024897965342,-16.7046695312708));
#8725=CARTESIAN_POINT('Ctrl Pts',(-13.5094758463079,41.2090214139111,-15.7960682062524));
#8726=CARTESIAN_POINT('Ctrl Pts',(-13.90040638973,40.8150808511182,-13.9221794105036));
#8727=CARTESIAN_POINT('Ctrl Pts',(-14.,40.7147688264544,-12.9568250138958));
#8728=CARTESIAN_POINT('Ctrl Pts',(-14.,40.7147688264544,-11.043174986104));
#8729=CARTESIAN_POINT('Ctrl Pts',(-13.90040638973,40.8150808511182,-10.0778205894962));
#8730=CARTESIAN_POINT('Ctrl Pts',(-13.5094758463079,41.2090214139111,-8.20393179374744));
#8731=CARTESIAN_POINT('Ctrl Pts',(-13.2182983629377,41.5024897965342,-7.29533046872903));
#8732=CARTESIAN_POINT('Ctrl Pts',(-12.116208359012,42.6142461507366,-4.74556937837981));
#8733=CARTESIAN_POINT('Ctrl Pts',(-11.0655427499361,43.6750742245956,-3.28315881526073));
#8734=CARTESIAN_POINT('Ctrl Pts',(-9.26451807446146,45.5025672498962,-1.45566578996008));
#8735=CARTESIAN_POINT('Ctrl Pts',(-8.49452237285655,46.2858563540338,-0.831293369425292));
#8736=CARTESIAN_POINT('Ctrl Pts',(-6.91295780738776,47.90695431736,0.210975884279631));
#8737=CARTESIAN_POINT('Ctrl Pts',(-6.10105549036537,48.7443794433284,0.628963504710973));
#8738=CARTESIAN_POINT('Ctrl Pts',(-4.53827705470841,50.3926460582921,1.27093230580056));
#8739=CARTESIAN_POINT('Ctrl Pts',(-3.78895528995956,51.194758981654,1.4947334563848));
#8740=CARTESIAN_POINT('Ctrl Pts',(-2.79295687688373,52.3791302063973,1.72280566002277));
#8741=CARTESIAN_POINT('Ctrl Pts',(-2.48603840542447,52.7631928777476,1.78012768145208));
#8742=CARTESIAN_POINT('Ctrl Pts',(-2.08733509638715,53.3786181712315,1.84417693298648));
#8743=CARTESIAN_POINT('Ctrl Pts',(-1.96562644092519,53.588391204841,1.86167854986234));
#8744=CARTESIAN_POINT('Ctrl Pts',(-1.76916191043536,54.05141346666,1.88812065613091));
#8745=CARTESIAN_POINT('Ctrl Pts',(-1.6909481438847,54.3031622530416,1.89750676829103));
#8746=CARTESIAN_POINT('Ctrl Pts',(-1.69094814388471,54.6122755947453,1.89750676829103));
#8747=CARTESIAN_POINT('',(1.69094814388473,54.6122755947453,1.89750676829103));
#8748=CARTESIAN_POINT('',(1.69094814388458,54.6122755947453,-25.8975067682909));
#8749=CARTESIAN_POINT('Ctrl Pts',(1.69094814388471,54.6122755947453,1.89750676829103));
#8750=CARTESIAN_POINT('Ctrl Pts',(1.6909481438847,54.3031622530416,1.89750676829103));
#8751=CARTESIAN_POINT('Ctrl Pts',(1.76916191043536,54.05141346666,1.88812065613091));
#8752=CARTESIAN_POINT('Ctrl Pts',(1.96562644092519,53.588391204841,1.86167854986234));
#8753=CARTESIAN_POINT('Ctrl Pts',(2.08733509638715,53.3786181712315,1.84417693298648));
#8754=CARTESIAN_POINT('Ctrl Pts',(2.48603840542448,52.7631928777475,1.78012768145208));
#8755=CARTESIAN_POINT('Ctrl Pts',(2.79295687688374,52.3791302063973,1.72280566002277));
#8756=CARTESIAN_POINT('Ctrl Pts',(3.78895528995957,51.194758981654,1.49473345638479));
#8757=CARTESIAN_POINT('Ctrl Pts',(4.53827705470842,50.3926460582921,1.27093230580055));
#8758=CARTESIAN_POINT('Ctrl Pts',(6.10105549036537,48.7443794433283,0.62896350471097));
#8759=CARTESIAN_POINT('Ctrl Pts',(6.91295780738778,47.90695431736,0.210975884279621));
#8760=CARTESIAN_POINT('Ctrl Pts',(8.49452237285656,46.2858563540338,-0.831293369425302));
#8761=CARTESIAN_POINT('Ctrl Pts',(9.26451807446146,45.5025672498962,-1.45566578996008));
#8762=CARTESIAN_POINT('Ctrl Pts',(11.0655427499361,43.6750742245956,-3.28315881526073));
#8763=CARTESIAN_POINT('Ctrl Pts',(12.116208359012,42.6142461507366,-4.74556937837981));
#8764=CARTESIAN_POINT('Ctrl Pts',(13.2182983629377,41.5024897965342,-7.29533046872903));
#8765=CARTESIAN_POINT('Ctrl Pts',(13.5094758463079,41.2090214139111,-8.20393179374743));
#8766=CARTESIAN_POINT('Ctrl Pts',(13.90040638973,40.8150808511182,-10.0778205894962));
#8767=CARTESIAN_POINT('Ctrl Pts',(14.,40.7147688264544,-11.043174986104));
#8768=CARTESIAN_POINT('Ctrl Pts',(14.,40.7147688264544,-12.9568250138958));
#8769=CARTESIAN_POINT('Ctrl Pts',(13.90040638973,40.8150808511182,-13.9221794105036));
#8770=CARTESIAN_POINT('Ctrl Pts',(13.5094758463079,41.2090214139111,-15.7960682062524));
#8771=CARTESIAN_POINT('Ctrl Pts',(13.2182983629377,41.5024897965342,-16.7046695312708));
#8772=CARTESIAN_POINT('Ctrl Pts',(12.116208359012,42.6142461507366,-19.25443062162));
#8773=CARTESIAN_POINT('Ctrl Pts',(11.0655427499361,43.6750742245956,-20.7168411847391));
#8774=CARTESIAN_POINT('Ctrl Pts',(9.26451807446145,45.5025672498962,-22.5443342100398));
#8775=CARTESIAN_POINT('Ctrl Pts',(8.49452237285654,46.2858563540338,-23.1687066305745));
#8776=CARTESIAN_POINT('Ctrl Pts',(6.91295780738774,47.90695431736,-24.2109758842795));
#8777=CARTESIAN_POINT('Ctrl Pts',(6.10105549036533,48.7443794433284,-24.6289635047108));
#8778=CARTESIAN_POINT('Ctrl Pts',(4.53827705470836,50.3926460582921,-25.2709323058004));
#8779=CARTESIAN_POINT('Ctrl Pts',(3.78895528995951,51.194758981654,-25.4947334563847));
#8780=CARTESIAN_POINT('Ctrl Pts',(2.79295687688367,52.3791302063973,-25.7228056600226));
#8781=CARTESIAN_POINT('Ctrl Pts',(2.48603840542441,52.7631928777475,-25.7801276814519));
#8782=CARTESIAN_POINT('Ctrl Pts',(2.08733509638707,53.3786181712314,-25.8441769329863));
#8783=CARTESIAN_POINT('Ctrl Pts',(1.9656264409251,53.588391204841,-25.8616785498622));
#8784=CARTESIAN_POINT('Ctrl Pts',(1.76916191043527,54.05141346666,-25.8881206561308));
#8785=CARTESIAN_POINT('Ctrl Pts',(1.69094814388459,54.3031622530415,-25.8975067682909));
#8786=CARTESIAN_POINT('Ctrl Pts',(1.69094814388459,54.6122755947453,-25.8975067682909));
#8787=CARTESIAN_POINT('Ctrl Pts',(1.69094814388459,54.6122755947453,-25.8975067682909));
#8788=CARTESIAN_POINT('Ctrl Pts',(1.69094814388459,54.9213889364491,-25.8975067682909));
#8789=CARTESIAN_POINT('Ctrl Pts',(1.76916191043525,55.1731377228307,-25.8881206561308));
#8790=CARTESIAN_POINT('Ctrl Pts',(1.9656264409251,55.6361599846497,-25.8616785498622));
#8791=CARTESIAN_POINT('Ctrl Pts',(2.0873350963871,55.8459330182592,-25.8441769329863));
#8792=CARTESIAN_POINT('Ctrl Pts',(2.48603840542444,56.4613583117431,-25.7801276814519));
#8793=CARTESIAN_POINT('Ctrl Pts',(2.79295687688369,56.8454209830934,-25.7228056600226));
#8794=CARTESIAN_POINT('Ctrl Pts',(3.78895528995954,58.0297922078367,-25.4947334563846));
#8795=CARTESIAN_POINT('Ctrl Pts',(4.53827705470839,58.8319051311986,-25.2709323058004));
#8796=CARTESIAN_POINT('Ctrl Pts',(6.10105549036536,60.4801717461623,-24.6289635047108));
#8797=CARTESIAN_POINT('Ctrl Pts',(6.91295780738777,61.3175968721307,-24.2109758842795));
#8798=CARTESIAN_POINT('Ctrl Pts',(8.49452237285657,62.9386948354569,-23.1687066305745));
#8799=CARTESIAN_POINT('Ctrl Pts',(9.26451807446147,63.7219839395945,-22.5443342100398));
#8800=CARTESIAN_POINT('Ctrl Pts',(11.0655427499361,65.5494769648951,-20.7168411847391));
#8801=CARTESIAN_POINT('Ctrl Pts',(12.116208359012,66.610305038754,-19.25443062162));
#8802=CARTESIAN_POINT('Ctrl Pts',(13.2182983629377,67.7220613929565,-16.7046695312708));
#8803=CARTESIAN_POINT('Ctrl Pts',(13.5094758463079,68.0155297755796,-15.7960682062524));
#8804=CARTESIAN_POINT('Ctrl Pts',(13.90040638973,68.4094703383725,-13.9221794105036));
#8805=CARTESIAN_POINT('Ctrl Pts',(14.,68.5097823630363,-12.9568250138958));
#8806=CARTESIAN_POINT('Ctrl Pts',(14.,68.5097823630363,-11.0431749861041));
#8807=CARTESIAN_POINT('Ctrl Pts',(13.90040638973,68.4094703383725,-10.0778205894963));
#8808=CARTESIAN_POINT('Ctrl Pts',(13.5094758463079,68.0155297755796,-8.20393179374744));
#8809=CARTESIAN_POINT('Ctrl Pts',(13.2182983629377,67.7220613929565,-7.29533046872904));
#8810=CARTESIAN_POINT('Ctrl Pts',(12.116208359012,66.610305038754,-4.74556937837982));
#8811=CARTESIAN_POINT('Ctrl Pts',(11.0655427499361,65.5494769648951,-3.28315881526074));
#8812=CARTESIAN_POINT('Ctrl Pts',(9.26451807446147,63.7219839395944,-1.45566578996009));
#8813=CARTESIAN_POINT('Ctrl Pts',(8.49452237285658,62.9386948354569,-0.831293369425317));
#8814=CARTESIAN_POINT('Ctrl Pts',(6.91295780738779,61.3175968721307,0.210975884279613));
#8815=CARTESIAN_POINT('Ctrl Pts',(6.10105549036539,60.4801717461623,0.628963504710959));
#8816=CARTESIAN_POINT('Ctrl Pts',(4.53827705470844,58.8319051311986,1.27093230580055));
#8817=CARTESIAN_POINT('Ctrl Pts',(3.78895528995959,58.0297922078367,1.49473345638479));
#8818=CARTESIAN_POINT('Ctrl Pts',(2.79295687688376,56.8454209830934,1.72280566002277));
#8819=CARTESIAN_POINT('Ctrl Pts',(2.4860384054245,56.4613583117431,1.78012768145208));
#8820=CARTESIAN_POINT('Ctrl Pts',(2.08733509638718,55.8459330182592,1.84417693298648));
#8821=CARTESIAN_POINT('Ctrl Pts',(1.96562644092521,55.6361599846497,1.86167854986234));
#8822=CARTESIAN_POINT('Ctrl Pts',(1.76916191043537,55.1731377228307,1.88812065613091));
#8823=CARTESIAN_POINT('Ctrl Pts',(1.6909481438847,54.9213889364491,1.89750676829103));
#8824=CARTESIAN_POINT('Ctrl Pts',(1.6909481438847,54.6122755947453,1.89750676829103));
#8825=CARTESIAN_POINT('Origin',(165.591979774207,54.6122755947453,-12.));
#8826=CARTESIAN_POINT('',(45.,54.6122755947453,-25.8975067682909));
#8827=CARTESIAN_POINT('Origin',(45.,54.6122755947453,-11.9999999999999));
#8828=CARTESIAN_POINT('',(165.591979774207,54.6122755947453,-25.8975067682909));
#8829=CARTESIAN_POINT('Origin',(5.94655548926424E-16,26.2427388041954,25.0000000000001));
#8830=CARTESIAN_POINT('',(-20.,72.1122755947453,-48.9999999999999));
#8831=CARTESIAN_POINT('',(-20.,72.1122755947453,-11.9999999999999));
#8832=CARTESIAN_POINT('',(-20.,72.1122755947453,-48.9999999999999));
#8833=CARTESIAN_POINT('',(-1.14423774522196E-16,76.2828667554667,-31.9999999999999));
#8834=CARTESIAN_POINT('Ctrl Pts',(1.38777878078145E-15,76.2828667554667,
-31.9999999999999));
#8835=CARTESIAN_POINT('Ctrl Pts',(-1.2705472609979,76.2828667554667,-31.9999999999999));
#8836=CARTESIAN_POINT('Ctrl Pts',(-2.58007773937013,76.2332652071209,-31.8769708923002));
#8837=CARTESIAN_POINT('Ctrl Pts',(-5.17618585589728,76.0314587231336,-31.3638289853873));
#8838=CARTESIAN_POINT('Ctrl Pts',(-6.46280366693617,75.8793792723685,-30.9738701002276));
#8839=CARTESIAN_POINT('Ctrl Pts',(-8.92278917996998,75.4966497262723,-29.9487995317102));
#8840=CARTESIAN_POINT('Ctrl Pts',(-10.0983665793023,75.2659618277825,-29.3128730480594));
#8841=CARTESIAN_POINT('Ctrl Pts',(-12.2682645673177,74.7684339328333,-27.8493616648039));
#8842=CARTESIAN_POINT('Ctrl Pts',(-13.2626071807075,74.5020216025358,-27.0216640667543));
#8843=CARTESIAN_POINT('Ctrl Pts',(-15.0225516277294,73.9834946181185,-25.2617196197324));
#8844=CARTESIAN_POINT('Ctrl Pts',(-15.8503625531969,73.7125357294074,-24.2669504874496));
#8845=CARTESIAN_POINT('Ctrl Pts',(-17.3134969066183,73.1986589652098,-22.0972715139887));
#8846=CARTESIAN_POINT('Ctrl Pts',(-17.9489707104667,72.9562551485406,-20.9223413606241));
#8847=CARTESIAN_POINT('Ctrl Pts',(-18.9735260730669,72.5495796554118,-18.4636662849712));
#8848=CARTESIAN_POINT('Ctrl Pts',(-19.363419845374,72.3854545732174,-17.1776933689394));
#8849=CARTESIAN_POINT('Ctrl Pts',(-19.876740954423,72.1666695578122,-14.5818027748883));
#8850=CARTESIAN_POINT('Ctrl Pts',(-20.,72.1122755947453,-13.2718294118763));
#8851=CARTESIAN_POINT('Ctrl Pts',(-20.,72.1122755947453,-11.9999999999999));
#8852=CARTESIAN_POINT('',(20.,72.1122755947453,-11.9999999999999));
#8853=CARTESIAN_POINT('Ctrl Pts',(20.,72.1122755947453,-11.9999999999999));
#8854=CARTESIAN_POINT('Ctrl Pts',(20.,72.1122755947453,-13.2718294118763));
#8855=CARTESIAN_POINT('Ctrl Pts',(19.876740954423,72.1666695578122,-14.5818027748883));
#8856=CARTESIAN_POINT('Ctrl Pts',(19.363419845374,72.3854545732174,-17.1776933689394));
#8857=CARTESIAN_POINT('Ctrl Pts',(18.9735260730669,72.5495796554118,-18.4636662849712));
#8858=CARTESIAN_POINT('Ctrl Pts',(17.9489707104667,72.9562551485406,-20.922341360624));
#8859=CARTESIAN_POINT('Ctrl Pts',(17.3134969066183,73.1986589652098,-22.0972715139887));
#8860=CARTESIAN_POINT('Ctrl Pts',(15.8503625531969,73.7125357294074,-24.2669504874496));
#8861=CARTESIAN_POINT('Ctrl Pts',(15.0225516277294,73.9834946181185,-25.2617196197324));
#8862=CARTESIAN_POINT('Ctrl Pts',(13.2626071807075,74.5020216025358,-27.0216640667543));
#8863=CARTESIAN_POINT('Ctrl Pts',(12.2682645673177,74.7684339328333,-27.8493616648039));
#8864=CARTESIAN_POINT('Ctrl Pts',(10.0983665793023,75.2659618277825,-29.3128730480594));
#8865=CARTESIAN_POINT('Ctrl Pts',(8.92278917996999,75.4966497262723,-29.9487995317102));
#8866=CARTESIAN_POINT('Ctrl Pts',(6.46280366693618,75.8793792723685,-30.9738701002276));
#8867=CARTESIAN_POINT('Ctrl Pts',(5.17618585589729,76.0314587231336,-31.3638289853873));
#8868=CARTESIAN_POINT('Ctrl Pts',(2.58007773937014,76.2332652071209,-31.8769708923002));
#8869=CARTESIAN_POINT('Ctrl Pts',(1.2705472609979,76.2828667554667,-31.9999999999999));
#8870=CARTESIAN_POINT('Ctrl Pts',(1.66533453693773E-15,76.2828667554667,
-31.9999999999999));
#8871=CARTESIAN_POINT('',(20.,72.1122755947453,-48.9999999999999));
#8872=CARTESIAN_POINT('',(20.,72.1122755947453,-48.9999999999999));
#8873=CARTESIAN_POINT('',(37.,59.9327136539873,-48.9999999999999));
#8874=CARTESIAN_POINT('Origin',(-1.31067715332243E-14,26.2427388041954,
-48.9999999999999));
#8875=CARTESIAN_POINT('',(37.,59.9327136539873,-58.9999999999999));
#8876=CARTESIAN_POINT('',(37.,59.9327136539873,-48.9999999999999));
#8877=CARTESIAN_POINT('',(-37.,59.9327136539873,-58.9999999999999));
#8878=CARTESIAN_POINT('Ctrl Pts',(-37.,59.9327136539873,-58.9999999999999));
#8879=CARTESIAN_POINT('Ctrl Pts',(-34.9241175691101,62.2125506169229,-58.9999999999999));
#8880=CARTESIAN_POINT('Ctrl Pts',(-32.5494800245177,64.3947066833499,-58.9999999999999));
#8881=CARTESIAN_POINT('Ctrl Pts',(-29.8860954400449,66.3779565652608,-58.9999999999999));
#8882=CARTESIAN_POINT('Ctrl Pts',(-27.222710855572,68.3612064471717,-58.9999999999999));
#8883=CARTESIAN_POINT('Ctrl Pts',(-24.2700583438171,70.1440603895185,-58.9999999999999));
#8884=CARTESIAN_POINT('Ctrl Pts',(-21.0832893198028,71.6245558330132,-58.9999999999999));
#8885=CARTESIAN_POINT('Ctrl Pts',(-17.8965202957886,73.105051276508,-58.9999999999999));
#8886=CARTESIAN_POINT('Ctrl Pts',(-14.4761422078645,74.2813950126213,-58.9999999999999));
#8887=CARTESIAN_POINT('Ctrl Pts',(-10.9229576299852,75.0761638529584,-58.9999999999999));
#8888=CARTESIAN_POINT('Ctrl Pts',(-7.36977305210587,75.8709326932955,-58.9999999999999));
#8889=CARTESIAN_POINT('Ctrl Pts',(-3.68542231180591,76.2828667554667,-58.9999999999999));
#8890=CARTESIAN_POINT('Ctrl Pts',(-8.60422844084496E-15,76.2828667554667,
-58.9999999999999));
#8891=CARTESIAN_POINT('Ctrl Pts',(3.68542231180589,76.2828667554668,-58.9999999999999));
#8892=CARTESIAN_POINT('Ctrl Pts',(7.36977305210586,75.8709326932955,-58.9999999999999));
#8893=CARTESIAN_POINT('Ctrl Pts',(10.9229576299852,75.0761638529584,-58.9999999999999));
#8894=CARTESIAN_POINT('Ctrl Pts',(14.4761422078645,74.2813950126214,-58.9999999999999));
#8895=CARTESIAN_POINT('Ctrl Pts',(17.8965202957886,73.105051276508,-58.9999999999999));
#8896=CARTESIAN_POINT('Ctrl Pts',(21.0832893198028,71.6245558330132,-58.9999999999999));
#8897=CARTESIAN_POINT('Ctrl Pts',(24.270058343817,70.1440603895185,-58.9999999999999));
#8898=CARTESIAN_POINT('Ctrl Pts',(27.222710855572,68.3612064471716,-58.9999999999999));
#8899=CARTESIAN_POINT('Ctrl Pts',(29.8860954400449,66.3779565652607,-58.9999999999999));
#8900=CARTESIAN_POINT('Ctrl Pts',(32.5494800245177,64.3947066833499,-58.9999999999999));
#8901=CARTESIAN_POINT('Ctrl Pts',(34.9241175691101,62.2125506169228,-58.9999999999999));
#8902=CARTESIAN_POINT('Ctrl Pts',(37.,59.9327136539873,-58.9999999999999));
#8903=CARTESIAN_POINT('',(-37.,59.9327136539873,-48.9999999999999));
#8904=CARTESIAN_POINT('',(-37.,59.9327136539873,-48.9999999999999));
#8905=CARTESIAN_POINT('Origin',(-1.31067715332243E-14,26.2427388041954,
-48.9999999999999));
#8906=CARTESIAN_POINT('Origin',(-99.7519848385422,5.,-11.9999999999999));
#8907=CARTESIAN_POINT('',(65.6680057154831,5.,25.0000000000001));
#8908=CARTESIAN_POINT('',(65.6680057154831,5.,-48.9999999999999));
#8909=CARTESIAN_POINT('',(65.6680057154831,5.,25.0000000000001));
#8910=CARTESIAN_POINT('',(125.680065601264,4.99999999999998,25.0000000000001));
#8911=CARTESIAN_POINT('',(65.6680057154831,5.,25.0000000000001));
#8912=CARTESIAN_POINT('',(125.680065601264,5.,35.0000000000001));
#8913=CARTESIAN_POINT('',(125.680065601264,5.,25.0000000000001));
#8914=CARTESIAN_POINT('',(145.859521458148,5.,35.0000000000001));
#8915=CARTESIAN_POINT('',(125.680065601264,5.,35.0000000000001));
#8916=CARTESIAN_POINT('',(145.859521458148,5.,-59.));
#8917=CARTESIAN_POINT('Origin',(99.7519848385422,5.,-11.9999999999999));
#8918=CARTESIAN_POINT('',(125.68006560189,4.99999999980207,-59.));
#8919=CARTESIAN_POINT('',(145.859521458148,5.,-58.9999999999999));
#8920=CARTESIAN_POINT('',(125.680065601265,4.99999999999999,-49.));
#8921=CARTESIAN_POINT('',(125.680065601265,5.,-49.));
#8922=CARTESIAN_POINT('',(65.6680057154831,5.,-48.9999999999999));
#8923=CARTESIAN_POINT('',(88.9375988864104,5.,-15.9999999999999));
#8924=CARTESIAN_POINT('Origin',(88.9375988864104,5.,-11.9999999999999));
#8925=CARTESIAN_POINT('',(115.629992744845,5.,-27.9631510575948));
#8926=CARTESIAN_POINT('Origin',(115.629992744845,5.,-11.9999999999999));
#8927=CARTESIAN_POINT('',(142.322386603279,5.,-15.9999999999999));
#8928=CARTESIAN_POINT('Origin',(142.322386603279,5.,-11.9999999999999));
#8929=CARTESIAN_POINT('Origin',(-85.4296283056384,23.8067054410607,25.0000000000001));
#8930=CARTESIAN_POINT('',(-37.,59.9327136539873,25.0000000000001));
#8931=CARTESIAN_POINT('',(-20.,72.1122755947453,25.0000000000001));
#8932=CARTESIAN_POINT('Origin',(5.94655548926424E-16,26.2427388041954,25.0000000000001));
#8933=CARTESIAN_POINT('',(-20.,-5.,25.0000000000001));
#8934=CARTESIAN_POINT('',(-65.6680057154831,-5.,25.0000000000001));
#8935=CARTESIAN_POINT('Ctrl Pts',(-125.680065601265,4.99999999999999,25.0000000000001));
#8936=CARTESIAN_POINT('Ctrl Pts',(-124.960945054864,5.22751276297754,25.0000000000001));
#8937=CARTESIAN_POINT('Ctrl Pts',(-124.243155867433,5.46012087178501,25.0000000000001));
#8938=CARTESIAN_POINT('Ctrl Pts',(-123.527427567709,5.69757964881347,25.0000000000001));
#8939=CARTESIAN_POINT('Ctrl Pts',(-122.804827886392,5.93731815946461,25.0000000000001));
#8940=CARTESIAN_POINT('Ctrl Pts',(-122.084328820779,6.18200089120545,25.0000000000001));
#8941=CARTESIAN_POINT('Ctrl Pts',(-121.366643614241,6.43133795177422,25.0000000000001));
#8942=CARTESIAN_POINT('Ctrl Pts',(-120.640583813992,6.68358450045882,25.0000000000001));
#8943=CARTESIAN_POINT('Ctrl Pts',(-119.91740388334,6.94059459252451,25.0000000000001));
#8944=CARTESIAN_POINT('Ctrl Pts',(-119.19780468018,7.20202979663394,25.0000000000001));
#8945=CARTESIAN_POINT('Ctrl Pts',(-118.46820637769,7.46709774041672,25.0000000000001));
#8946=CARTESIAN_POINT('Ctrl Pts',(-117.742288953963,7.73671457758463,25.0000000000001));
#8947=CARTESIAN_POINT('Ctrl Pts',(-117.020745101533,8.01048912839484,25.0000000000001));
#8948=CARTESIAN_POINT('Ctrl Pts',(-116.287407035734,8.28873874396535,25.0000000000001));
#8949=CARTESIAN_POINT('Ctrl Pts',(-115.558586627373,8.57128304592011,25.0000000000001));
#8950=CARTESIAN_POINT('Ctrl Pts',(-114.834973164448,8.85767273946868,25.0000000000001));
#8951=CARTESIAN_POINT('Ctrl Pts',(-114.357879489923,9.0464955271055,25.0000000000001));
#8952=CARTESIAN_POINT('Ctrl Pts',(-113.883048517548,9.23698912926061,25.0000000000001));
#8953=CARTESIAN_POINT('Ctrl Pts',(-113.410669261531,9.42901606958512,25.0000000000001));
#8954=CARTESIAN_POINT('Ctrl Pts',(-113.363716076149,9.44810301384167,25.0000000000001));
#8955=CARTESIAN_POINT('Ctrl Pts',(-113.316778572265,9.46720857102223,25.0000000000001));
#8956=CARTESIAN_POINT('Ctrl Pts',(-113.269855341093,9.48633327990069,25.0000000000001));
#8957=CARTESIAN_POINT('Ctrl Pts',(-112.214947248068,9.91628683741896,25.0000000000001));
#8958=CARTESIAN_POINT('Ctrl Pts',(-111.167493669256,10.3558266948226,25.0000000000001));
#8959=CARTESIAN_POINT('Ctrl Pts',(-110.127707792712,10.804452542433,25.0000000000001));
#8960=CARTESIAN_POINT('Ctrl Pts',(-109.064746553832,11.2630776281616,25.0000000000001));
#8961=CARTESIAN_POINT('Ctrl Pts',(-108.00979854462,11.7311981609204,25.0000000000001));
#8962=CARTESIAN_POINT('Ctrl Pts',(-106.963052490346,12.2082398956616,25.0000000000001));
#8963=CARTESIAN_POINT('Ctrl Pts',(-105.889281591192,12.6975978735168,25.0000000000001));
#8964=CARTESIAN_POINT('Ctrl Pts',(-104.824141527827,13.1963435545408,25.0000000000001));
#8965=CARTESIAN_POINT('Ctrl Pts',(-103.76779680625,13.7038170919497,25.0000000000001));
#8966=CARTESIAN_POINT('Ctrl Pts',(-102.679455390731,14.2266620087278,25.0000000000001));
#8967=CARTESIAN_POINT('Ctrl Pts',(-101.600450087039,14.7587714042181,25.0000000000001));
#8968=CARTESIAN_POINT('Ctrl Pts',(-100.530921385051,15.2993833950381,25.0000000000001));
#8969=CARTESIAN_POINT('Ctrl Pts',(-100.159757279432,15.4869947846971,25.0000000000001));
#8970=CARTESIAN_POINT('Ctrl Pts',(-99.7897341428704,15.6756298332555,25.0000000000001));
#8971=CARTESIAN_POINT('Ctrl Pts',(-99.4208568320684,15.8652556601936,25.0000000000001));
#8972=CARTESIAN_POINT('Ctrl Pts',(-99.2980442797775,15.928388932706,25.0000000000001));
#8973=CARTESIAN_POINT('Ctrl Pts',(-99.1753587340892,15.9916320252805,25.0000000000001));
#8974=CARTESIAN_POINT('Ctrl Pts',(-99.0528003622234,16.054983712168,25.0000000000001));
#8975=CARTESIAN_POINT('Ctrl Pts',(-98.9807005502699,16.0922528488413,25.0000000000001));
#8976=CARTESIAN_POINT('Ctrl Pts',(-98.9086371756676,16.1295634823898,25.0000000000001));
#8977=CARTESIAN_POINT('Ctrl Pts',(-98.8366072848604,16.1669169540907,25.0000000000001));
#8978=CARTESIAN_POINT('Ctrl Pts',(-97.8146405969214,16.6968914317609,25.0000000000001));
#8979=CARTESIAN_POINT('Ctrl Pts',(-96.7996148754077,17.235390438076,25.0000000000001));
#8980=CARTESIAN_POINT('Ctrl Pts',(-95.7917345876971,17.7817475522874,25.0000000000001));
#8981=CARTESIAN_POINT('Ctrl Pts',(-94.7526454700998,18.3450225152184,25.0000000000001));
#8982=CARTESIAN_POINT('Ctrl Pts',(-93.7211510251918,18.9166496466945,25.0000000000001));
#8983=CARTESIAN_POINT('Ctrl Pts',(-92.6974362009878,19.4958587242714,25.0000000000001));
#8984=CARTESIAN_POINT('Ctrl Pts',(-91.6354743167707,20.0967076607488,25.0000000000001));
#8985=CARTESIAN_POINT('Ctrl Pts',(-90.5818840659185,20.7057155131889,25.0000000000001));
#8986=CARTESIAN_POINT('Ctrl Pts',(-89.5368325915886,21.3219821917453,25.0000000000001));
#8987=CARTESIAN_POINT('Ctrl Pts',(-88.4432597431563,21.9668619164451,25.0000000000001));
#8988=CARTESIAN_POINT('Ctrl Pts',(-87.3590367834119,22.6196899704338,25.0000000000001));
#8989=CARTESIAN_POINT('Ctrl Pts',(-86.2843156503055,23.2793942945683,25.0000000000001));
#8990=CARTESIAN_POINT('Ctrl Pts',(-86.1473152047691,23.363490329851,25.0000000000001));
#8991=CARTESIAN_POINT('Ctrl Pts',(-86.0104691157456,23.4476980549826,25.0000000000001));
#8992=CARTESIAN_POINT('Ctrl Pts',(-85.8737776574015,23.5320152073781,25.0000000000001));
#8993=CARTESIAN_POINT('Ctrl Pts',(-85.808653088074,23.5721868340709,25.0000000000001));
#8994=CARTESIAN_POINT('Ctrl Pts',(-85.7435636182602,23.6123832995439,25.0000000000001));
#8995=CARTESIAN_POINT('Ctrl Pts',(-85.6785092769395,23.6526043584145,25.0000000000001));
#8996=CARTESIAN_POINT('Ctrl Pts',(-85.6271072730019,23.6843846052738,25.0000000000001));
#8997=CARTESIAN_POINT('Ctrl Pts',(-85.575725209178,23.716181433953,25.0000000000001));
#8998=CARTESIAN_POINT('Ctrl Pts',(-85.5243537468771,23.748000533409,25.0000000000001));
#8999=CARTESIAN_POINT('Ctrl Pts',(-84.6574156247278,24.2849755209869,25.0000000000001));
#9000=CARTESIAN_POINT('Ctrl Pts',(-83.7942589216096,24.8278271617857,25.0000000000001));
#9001=CARTESIAN_POINT('Ctrl Pts',(-82.9353696413023,25.3758221435343,25.0000000000001));
#9002=CARTESIAN_POINT('Ctrl Pts',(-82.045861072411,25.9433530734819,25.0000000000001));
#9003=CARTESIAN_POINT('Ctrl Pts',(-81.1609294663116,26.5164004546283,25.0000000000001));
#9004=CARTESIAN_POINT('Ctrl Pts',(-80.2810757074104,27.0941097060007,25.0000000000001));
#9005=CARTESIAN_POINT('Ctrl Pts',(-79.3348226214597,27.715416549738,25.0000000000001));
#9006=CARTESIAN_POINT('Ctrl Pts',(-78.3944426985011,28.3421154388075,25.0000000000001));
#9007=CARTESIAN_POINT('Ctrl Pts',(-77.4605156372659,28.9730986607385,25.0000000000001));
#9008=CARTESIAN_POINT('Ctrl Pts',(-76.5849590173578,29.5646454312988,25.0000000000001));
#9009=CARTESIAN_POINT('Ctrl Pts',(-75.715073061572,30.159956917886,25.0000000000001));
#9010=CARTESIAN_POINT('Ctrl Pts',(-74.8513063154526,30.7580902197078,25.0000000000001));
#9011=CARTESIAN_POINT('Ctrl Pts',(-74.4464156532091,31.0384652049367,25.0000000000001));
#9012=CARTESIAN_POINT('Ctrl Pts',(-74.042869183162,31.3194598427701,25.0000000000001));
#9013=CARTESIAN_POINT('Ctrl Pts',(-73.6407113925489,31.600975230648,25.0000000000001));
#9014=CARTESIAN_POINT('Ctrl Pts',(-73.5345264758602,31.6753059752118,25.0000000000001));
#9015=CARTESIAN_POINT('Ctrl Pts',(-73.4284383672046,31.7496730189567,25.0000000000001));
#9016=CARTESIAN_POINT('Ctrl Pts',(-73.3224478746784,31.824074529959,25.0000000000001));
#9017=CARTESIAN_POINT('Ctrl Pts',(-73.2658918473683,31.8637748255974,25.0000000000001));
#9018=CARTESIAN_POINT('Ctrl Pts',(-73.2093636136334,31.9034849348122,25.0000000000001));
#9019=CARTESIAN_POINT('Ctrl Pts',(-73.1528632957563,31.9432045787683,25.0000000000001));
#9020=CARTESIAN_POINT('Ctrl Pts',(-73.1171533786224,31.9683086002598,25.0000000000001));
#9021=CARTESIAN_POINT('Ctrl Pts',(-73.0814546128172,31.9934164305148,25.0000000000001));
#9022=CARTESIAN_POINT('Ctrl Pts',(-73.0457670291454,32.0185279990633,25.0000000000001));
#9023=CARTESIAN_POINT('Ctrl Pts',(-73.0063553520497,32.0462600259806,25.0000000000001));
#9024=CARTESIAN_POINT('Ctrl Pts',(-72.9669507059342,32.0740012593469,25.0000000000001));
#9025=CARTESIAN_POINT('Ctrl Pts',(-72.9275465923938,32.1017562294851,25.0000000000001));
#9026=CARTESIAN_POINT('Ctrl Pts',(-71.754282216512,32.9281653221144,25.0000000000001));
#9027=CARTESIAN_POINT('Ctrl Pts',(-70.5832630059994,33.765499217731,25.0000000000001));
#9028=CARTESIAN_POINT('Ctrl Pts',(-69.4119648391555,34.6144663184202,25.0000000000001));
#9029=CARTESIAN_POINT('Ctrl Pts',(-67.5244483181643,35.9825547127243,25.0000000000001));
#9030=CARTESIAN_POINT('Ctrl Pts',(-65.6362106229917,37.3808549641196,25.0000000000001));
#9031=CARTESIAN_POINT('Ctrl Pts',(-63.736803082023,38.8124625160226,25.0000000000001));
#9032=CARTESIAN_POINT('Ctrl Pts',(-63.1641508526633,39.244077763663,25.0000000000001));
#9033=CARTESIAN_POINT('Ctrl Pts',(-62.5904834077693,39.6787207396113,25.0000000000001));
#9034=CARTESIAN_POINT('Ctrl Pts',(-62.015513259775,40.1164754881207,25.0000000000001));
#9035=CARTESIAN_POINT('Ctrl Pts',(-61.7459960029027,40.3216730264845,25.0000000000001));
#9036=CARTESIAN_POINT('Ctrl Pts',(-61.4761924871871,40.5275542859727,25.0000000000001));
#9037=CARTESIAN_POINT('Ctrl Pts',(-61.2060729689618,40.7341278022368,25.0000000000001));
#9038=CARTESIAN_POINT('Ctrl Pts',(-61.1367061914413,40.7871759464008,25.0000000000001));
#9039=CARTESIAN_POINT('Ctrl Pts',(-61.0673185741674,40.8402697419253,25.0000000000001));
#9040=CARTESIAN_POINT('Ctrl Pts',(-60.9979096122979,40.8934093323168,25.0000000000001));
#9041=CARTESIAN_POINT('Ctrl Pts',(-60.9490449425875,40.9308201862337,25.0000000000001));
#9042=CARTESIAN_POINT('Ctrl Pts',(-60.9001696938147,40.9682537375167,25.0000000000001));
#9043=CARTESIAN_POINT('Ctrl Pts',(-60.8512836896761,41.0057100361011,25.0000000000001));
#9044=CARTESIAN_POINT('Ctrl Pts',(-60.8325758368311,41.0200439325687,25.0000000000001));
#9045=CARTESIAN_POINT('Ctrl Pts',(-60.8138664088997,41.0343811602963,25.0000000000001));
#9046=CARTESIAN_POINT('Ctrl Pts',(-60.7951553959967,41.0487217220779,25.0000000000001));
#9047=CARTESIAN_POINT('Ctrl Pts',(-60.7754197597175,41.0638475793912,25.0000000000001));
#9048=CARTESIAN_POINT('Ctrl Pts',(-60.7556889733333,41.0789720776831,25.0000000000001));
#9049=CARTESIAN_POINT('Ctrl Pts',(-60.7359667875713,41.0940923301713,25.0000000000001));
#9050=CARTESIAN_POINT('Ctrl Pts',(-60.0445237146081,41.6241955332639,25.0000000000001));
#9051=CARTESIAN_POINT('Ctrl Pts',(-59.3621639470488,42.1502148040397,25.0000000000001));
#9052=CARTESIAN_POINT('Ctrl Pts',(-58.6878564666335,42.6724517572262,25.0000000000001));
#9053=CARTESIAN_POINT('Ctrl Pts',(-57.9873078541347,43.2150119149827,25.0000000000001));
#9054=CARTESIAN_POINT('Ctrl Pts',(-57.2954506251931,43.7534898234267,25.0000000000001));
#9055=CARTESIAN_POINT('Ctrl Pts',(-56.6111684755191,44.288264626604,25.0000000000001));
#9056=CARTESIAN_POINT('Ctrl Pts',(-56.205629463576,44.6051982853235,25.0000000000001));
#9057=CARTESIAN_POINT('Ctrl Pts',(-55.8027518035775,44.9208320505127,25.0000000000001));
#9058=CARTESIAN_POINT('Ctrl Pts',(-55.4023089152689,45.2352508066007,25.0000000000001));
#9059=CARTESIAN_POINT('Ctrl Pts',(-55.2146013113743,45.3826345985169,25.0000000000001));
#9060=CARTESIAN_POINT('Ctrl Pts',(-55.0274287488623,45.529751479852,25.0000000000001));
#9061=CARTESIAN_POINT('Ctrl Pts',(-54.8407681811854,45.6766104934432,25.0000000000001));
#9062=CARTESIAN_POINT('Ctrl Pts',(-54.8222267879297,45.6911983132384,25.0000000000001));
#9063=CARTESIAN_POINT('Ctrl Pts',(-54.8036903862308,45.7057836357621,25.0000000000001));
#9064=CARTESIAN_POINT('Ctrl Pts',(-54.7851477621434,45.7203752785472,25.0000000000001));
#9065=CARTESIAN_POINT('Ctrl Pts',(-54.3014372043673,46.1010189046712,25.0000000000001));
#9066=CARTESIAN_POINT('Ctrl Pts',(-53.815452761034,46.4844273276019,25.0000000000001));
#9067=CARTESIAN_POINT('Ctrl Pts',(-53.3318153552279,46.8668393594794,25.0000000000001));
#9068=CARTESIAN_POINT('Ctrl Pts',(-52.793096355682,47.2928044001363,25.0000000000001));
#9069=CARTESIAN_POINT('Ctrl Pts',(-52.2572888932505,47.7175326831695,25.0000000000001));
#9070=CARTESIAN_POINT('Ctrl Pts',(-51.7307337221954,48.1357755371239,25.0000000000001));
#9071=CARTESIAN_POINT('Ctrl Pts',(-51.1509899550892,48.5962661011628,25.0000000000001));
#9072=CARTESIAN_POINT('Ctrl Pts',(-50.5824604036283,49.0488932231173,25.0000000000001));
#9073=CARTESIAN_POINT('Ctrl Pts',(-50.033573635379,49.4866107010153,25.0000000000001));
#9074=CARTESIAN_POINT('Ctrl Pts',(-49.7934356742699,49.6781120975957,25.0000000000001));
#9075=CARTESIAN_POINT('Ctrl Pts',(-49.5570572165051,49.8667593624178,25.0000000000001));
#9076=CARTESIAN_POINT('Ctrl Pts',(-49.3251436624354,50.051961667685,25.0000000000001));
#9077=CARTESIAN_POINT('Ctrl Pts',(-49.2979662928179,50.0736650628335,25.0000000000001));
#9078=CARTESIAN_POINT('Ctrl Pts',(-49.2708502396166,50.0953211487278,25.0000000000001));
#9079=CARTESIAN_POINT('Ctrl Pts',(-49.243796638345,50.116928974649,25.0000000000001));
#9080=CARTESIAN_POINT('Ctrl Pts',(-49.2360887390484,50.1230853064641,25.0000000000001));
#9081=CARTESIAN_POINT('Ctrl Pts',(-49.2283859092831,50.1292377207798,25.0000000000001));
#9082=CARTESIAN_POINT('Ctrl Pts',(-49.2206881753122,50.135386195609,25.0000000000001));
#9083=CARTESIAN_POINT('Ctrl Pts',(-49.2136388166439,50.1410167882612,25.0000000000001));
#9084=CARTESIAN_POINT('Ctrl Pts',(-49.2065859857244,50.1466502639488,25.0000000000001));
#9085=CARTESIAN_POINT('Ctrl Pts',(-49.1995286205646,50.1522874709358,25.0000000000001));
#9086=CARTESIAN_POINT('Ctrl Pts',(-48.5736996895669,50.6521804398544,25.0000000000001));
#9087=CARTESIAN_POINT('Ctrl Pts',(-47.9148954411139,51.1792736794625,25.0000000000001));
#9088=CARTESIAN_POINT('Ctrl Pts',(-47.2031261108418,51.7495555800309,25.0000000000001));
#9089=CARTESIAN_POINT('Ctrl Pts',(-46.7322561076265,52.1268247723569,25.0000000000001));
#9090=CARTESIAN_POINT('Ctrl Pts',(-46.2382071196254,52.5229967428189,25.0000000000001));
#9091=CARTESIAN_POINT('Ctrl Pts',(-45.7151727286514,52.9426877028818,25.0000000000001));
#9092=CARTESIAN_POINT('Ctrl Pts',(-45.2673909231485,53.3019948136441,25.0000000000001));
#9093=CARTESIAN_POINT('Ctrl Pts',(-44.7983649128932,53.6785406963364,25.0000000000001));
#9094=CARTESIAN_POINT('Ctrl Pts',(-44.3044261761361,54.0752003649523,25.0000000000001));
#9095=CARTESIAN_POINT('Ctrl Pts',(-43.9514920159341,54.35862569002,25.0000000000001));
#9096=CARTESIAN_POINT('Ctrl Pts',(-43.5858381908448,54.6523198557899,25.0000000000001));
#9097=CARTESIAN_POINT('Ctrl Pts',(-43.2061138913264,54.9573203095084,25.0000000000001));
#9098=CARTESIAN_POINT('Ctrl Pts',(-43.1230492008067,55.0240391587593,25.0000000000001));
#9099=CARTESIAN_POINT('Ctrl Pts',(-43.0393111656161,55.0912989849344,25.0000000000001));
#9100=CARTESIAN_POINT('Ctrl Pts',(-42.9548855554703,55.159110563518,25.0000000000001));
#9101=CARTESIAN_POINT('Ctrl Pts',(-42.9487467129319,55.16404134936,25.0000000000001));
#9102=CARTESIAN_POINT('Ctrl Pts',(-42.9426034491638,55.1689756836288,25.0000000000001));
#9103=CARTESIAN_POINT('Ctrl Pts',(-42.9364581930475,55.1739116151576,25.0000000000001));
#9104=CARTESIAN_POINT('Ctrl Pts',(-42.4342170449237,55.5773167574626,25.0000000000001));
#9105=CARTESIAN_POINT('Ctrl Pts',(-41.956235985396,55.9612098550919,25.0000000000001));
#9106=CARTESIAN_POINT('Ctrl Pts',(-41.5020206332019,56.3258915173201,25.0000000000001));
#9107=CARTESIAN_POINT('Ctrl Pts',(-40.9919258908233,56.735437776921,25.0000000000001));
#9108=CARTESIAN_POINT('Ctrl Pts',(-40.5118042106407,57.1207550280515,25.0000000000001));
#9109=CARTESIAN_POINT('Ctrl Pts',(-40.0610034128949,57.4823195544779,25.0000000000001));
#9110=CARTESIAN_POINT('Ctrl Pts',(-39.5686598282259,57.8772034498039,25.0000000000001));
#9111=CARTESIAN_POINT('Ctrl Pts',(-39.1112908860053,58.2437558219308,25.0000000000001));
#9112=CARTESIAN_POINT('Ctrl Pts',(-38.6880935424586,58.5826469939407,25.0000000000001));
#9113=CARTESIAN_POINT('Ctrl Pts',(-38.1712113731884,58.9965598098081,25.0000000000001));
#9114=CARTESIAN_POINT('Ctrl Pts',(-37.7053057014659,59.3692096416051,25.0000000000001));
#9115=CARTESIAN_POINT('Ctrl Pts',(-37.2889677026751,59.7018784459919,25.0000000000001));
#9116=CARTESIAN_POINT('Ctrl Pts',(-37.1898413829962,59.7810838856746,25.0000000000001));
#9117=CARTESIAN_POINT('Ctrl Pts',(-37.0935250781658,59.8580230943006,25.0000000000001));
#9118=CARTESIAN_POINT('Ctrl Pts',(-37.,59.9327136539873,25.0000000000001));
#9119=CARTESIAN_POINT('Origin',(-85.4296283056384,23.8067054410607,25.0000000000001));
#9120=CARTESIAN_POINT('',(65.6680057154831,-5.,25.0000000000001));
#9121=CARTESIAN_POINT('',(20.,72.1122755947453,25.0000000000001));
#9122=CARTESIAN_POINT('',(20.,72.1122755947453,25.0000000000001));
#9123=CARTESIAN_POINT('',(37.,59.9327136539873,25.0000000000001));
#9124=CARTESIAN_POINT('Origin',(5.94655548926424E-16,26.2427388041954,25.0000000000001));
#9125=CARTESIAN_POINT('Ctrl Pts',(37.,59.9327136539873,25.0000000000001));
#9126=CARTESIAN_POINT('Ctrl Pts',(37.379667023306,59.6295057548716,25.0000000000001));
#9127=CARTESIAN_POINT('Ctrl Pts',(37.8053353012187,59.2892352085535,25.0000000000001));
#9128=CARTESIAN_POINT('Ctrl Pts',(38.2782656703118,58.9107382150177,25.0000000000001));
#9129=CARTESIAN_POINT('Ctrl Pts',(38.6687156895296,58.5982521323764,25.0000000000001));
#9130=CARTESIAN_POINT('Ctrl Pts',(39.0913794549942,58.2597099653507,25.0000000000001));
#9131=CARTESIAN_POINT('Ctrl Pts',(39.5469874492648,57.8944807883205,25.0000000000001));
#9132=CARTESIAN_POINT('Ctrl Pts',(39.9543075803571,57.5679606259497,25.0000000000001));
#9133=CARTESIAN_POINT('Ctrl Pts',(40.3879583984683,57.2201102048173,25.0000000000001));
#9134=CARTESIAN_POINT('Ctrl Pts',(40.8484865188096,56.8505053738539,25.0000000000001));
#9135=CARTESIAN_POINT('Ctrl Pts',(41.2999783576224,56.4881527673678,25.0000000000001));
#9136=CARTESIAN_POINT('Ctrl Pts',(41.777302381718,56.1048903670244,25.0000000000001));
#9137=CARTESIAN_POINT('Ctrl Pts',(42.2810069638633,55.7003537526117,25.0000000000001));
#9138=CARTESIAN_POINT('Ctrl Pts',(42.4049655133756,55.6007998201585,25.0000000000001));
#9139=CARTESIAN_POINT('Ctrl Pts',(42.5305219159893,55.4999576756661,25.0000000000001));
#9140=CARTESIAN_POINT('Ctrl Pts',(42.6576847433865,55.3978223055861,25.0000000000001));
#9141=CARTESIAN_POINT('Ctrl Pts',(42.7210177921879,55.3469541036908,25.0000000000001));
#9142=CARTESIAN_POINT('Ctrl Pts',(42.7847493184706,55.2957651191222,25.0000000000001));
#9143=CARTESIAN_POINT('Ctrl Pts',(42.8488803978488,55.2442547498818,25.0000000000001));
#9144=CARTESIAN_POINT('Ctrl Pts',(42.8670093092844,55.2296935272885,25.0000000000001));
#9145=CARTESIAN_POINT('Ctrl Pts',(42.885170149462,55.21510662261,25.0000000000001));
#9146=CARTESIAN_POINT('Ctrl Pts',(42.9033629428465,55.2004940224215,25.0000000000001));
#9147=CARTESIAN_POINT('Ctrl Pts',(42.9117835396531,55.1937305303132,25.0000000000001));
#9148=CARTESIAN_POINT('Ctrl Pts',(42.9202109819016,55.1869615333721,25.0000000000001));
#9149=CARTESIAN_POINT('Ctrl Pts',(42.9286452720233,55.1801870302728,25.0000000000001));
#9150=CARTESIAN_POINT('Ctrl Pts',(42.9355167001405,55.1746678329952,25.0000000000001));
#9151=CARTESIAN_POINT('Ctrl Pts',(42.9423940941063,55.169143839983,25.0000000000001));
#9152=CARTESIAN_POINT('Ctrl Pts',(42.949264125121,55.1636257574225,25.0000000000001));
#9153=CARTESIAN_POINT('Ctrl Pts',(43.4538066664403,54.7583717793348,25.0000000000001));
#9154=CARTESIAN_POINT('Ctrl Pts',(43.9338047887228,54.3728188661298,25.0000000000001));
#9155=CARTESIAN_POINT('Ctrl Pts',(44.3922742549877,54.0046546909899,25.0000000000001));
#9156=CARTESIAN_POINT('Ctrl Pts',(44.9182289894069,53.5822979034466,25.0000000000001));
#9157=CARTESIAN_POINT('Ctrl Pts',(45.4158501546012,53.1828251430864,25.0000000000001));
#9158=CARTESIAN_POINT('Ctrl Pts',(45.8896418211895,52.8027007016266,25.0000000000001));
#9159=CARTESIAN_POINT('Ctrl Pts',(46.5104671522248,52.3046107206372,25.0000000000001));
#9160=CARTESIAN_POINT('Ctrl Pts',(47.0903771812918,51.8397403801932,25.0000000000001));
#9161=CARTESIAN_POINT('Ctrl Pts',(47.6394345771857,51.4000748549018,25.0000000000001));
#9162=CARTESIAN_POINT('Ctrl Pts',(47.9907462386239,51.1187570412772,25.0000000000001));
#9163=CARTESIAN_POINT('Ctrl Pts',(48.3294254446928,50.8477570196711,25.0000000000001));
#9164=CARTESIAN_POINT('Ctrl Pts',(48.6581018226499,50.5849711025823,25.0000000000001));
#9165=CARTESIAN_POINT('Ctrl Pts',(48.8198722274257,50.4556311590152,25.0000000000001));
#9166=CARTESIAN_POINT('Ctrl Pts',(48.9792194319725,50.3282810641903,25.0000000000001));
#9167=CARTESIAN_POINT('Ctrl Pts',(49.1364569454656,50.2026700971239,25.0000000000001));
#9168=CARTESIAN_POINT('Ctrl Pts',(49.1559822657899,50.1870720740203,25.0000000000001));
#9169=CARTESIAN_POINT('Ctrl Pts',(49.1754750548033,50.1715008684445,25.0000000000001));
#9170=CARTESIAN_POINT('Ctrl Pts',(49.194935912914,50.1559560004978,25.0000000000001));
#9171=CARTESIAN_POINT('Ctrl Pts',(49.2026425963922,50.1498000860826,25.0000000000001));
#9172=CARTESIAN_POINT('Ctrl Pts',(49.2103442723557,50.1436483020264,25.0000000000001));
#9173=CARTESIAN_POINT('Ctrl Pts',(49.2180409780931,50.1375006185279,25.0000000000001));
#9174=CARTESIAN_POINT('Ctrl Pts',(49.2253110938493,50.1316936704398,25.0000000000001));
#9175=CARTESIAN_POINT('Ctrl Pts',(49.2325829791765,50.1258854254269,25.0000000000001));
#9176=CARTESIAN_POINT('Ctrl Pts',(49.2398606897643,50.1200726448833,25.0000000000001));
#9177=CARTESIAN_POINT('Ctrl Pts',(49.8606042856743,49.6242785001005,25.0000000000001));
#9178=CARTESIAN_POINT('Ctrl Pts',(50.5142825462621,49.1030328807307,25.0000000000001));
#9179=CARTESIAN_POINT('Ctrl Pts',(51.1871655721719,48.567830362299,25.0000000000001));
#9180=CARTESIAN_POINT('Ctrl Pts',(51.7158663366829,48.1473085631639,25.0000000000001));
#9181=CARTESIAN_POINT('Ctrl Pts',(52.2564249707963,47.7181716623712,25.0000000000001));
#9182=CARTESIAN_POINT('Ctrl Pts',(52.8021626903985,47.2859712302726,25.0000000000001));
#9183=CARTESIAN_POINT('Ctrl Pts',(53.2807819115689,46.9069257167037,25.0000000000001));
#9184=CARTESIAN_POINT('Ctrl Pts',(53.7633851027738,46.5255242814923,25.0000000000001));
#9185=CARTESIAN_POINT('Ctrl Pts',(54.2454397069039,46.1454810332774,25.0000000000001));
#9186=CARTESIAN_POINT('Ctrl Pts',(54.4068021109733,46.0182657932259,25.0000000000001));
#9187=CARTESIAN_POINT('Ctrl Pts',(54.5681027698807,45.8912024350973,25.0000000000001));
#9188=CARTESIAN_POINT('Ctrl Pts',(54.729170760509,45.7644292654329,25.0000000000001));
#9189=CARTESIAN_POINT('Ctrl Pts',(54.7576244445241,45.7420339794598,25.0000000000001));
#9190=CARTESIAN_POINT('Ctrl Pts',(54.7860708662357,45.7196477481137,25.0000000000001));
#9191=CARTESIAN_POINT('Ctrl Pts',(54.8145090816246,45.6972713320229,25.0000000000001));
#9192=CARTESIAN_POINT('Ctrl Pts',(54.8348702776094,45.6812502636389,25.0000000000001));
#9193=CARTESIAN_POINT('Ctrl Pts',(54.8552330883136,45.6652296458008,25.0000000000001));
#9194=CARTESIAN_POINT('Ctrl Pts',(54.8756040257786,45.6492043660801,25.0000000000001));
#9195=CARTESIAN_POINT('Ctrl Pts',(55.5550265500445,45.1147205693163,25.0000000000001));
#9196=CARTESIAN_POINT('Ctrl Pts',(56.2412452453015,44.5768116431681,25.0000000000001));
#9197=CARTESIAN_POINT('Ctrl Pts',(56.9353824441227,44.0350550110448,25.0000000000001));
#9198=CARTESIAN_POINT('Ctrl Pts',(57.5651721195718,43.5435200031287,25.0000000000001));
#9199=CARTESIAN_POINT('Ctrl Pts',(58.2014803619766,43.048817738353,25.0000000000001));
#9200=CARTESIAN_POINT('Ctrl Pts',(58.8451714214353,42.5506593941846,25.0000000000001));
#9201=CARTESIAN_POINT('Ctrl Pts',(59.4687471352858,42.0680684982715,25.0000000000001));
#9202=CARTESIAN_POINT('Ctrl Pts',(60.0992513234504,41.5822340273024,25.0000000000001));
#9203=CARTESIAN_POINT('Ctrl Pts',(60.7374957459951,41.0929201403882,25.0000000000001));
#9204=CARTESIAN_POINT('Ctrl Pts',(60.7575133230696,41.0775735457312,25.0000000000001));
#9205=CARTESIAN_POINT('Ctrl Pts',(60.7775403998995,41.0622220872218,25.0000000000001));
#9206=CARTESIAN_POINT('Ctrl Pts',(60.7975709297175,41.0468704118127,25.0000000000001));
#9207=CARTESIAN_POINT('Ctrl Pts',(62.1358201086493,40.0212177107564,25.0000000000001));
#9208=CARTESIAN_POINT('Ctrl Pts',(63.4659680993238,39.012623086552,25.0000000000001));
#9209=CARTESIAN_POINT('Ctrl Pts',(64.791604272834,38.0200398160107,25.0000000000001));
#9210=CARTESIAN_POINT('Ctrl Pts',(66.1951427752259,36.9691264018528,25.0000000000001));
#9211=CARTESIAN_POINT('Ctrl Pts',(67.5936194820664,35.9361573083481,25.0000000000001));
#9212=CARTESIAN_POINT('Ctrl Pts',(68.9912744880311,34.9198762099585,25.0000000000001));
#9213=CARTESIAN_POINT('Ctrl Pts',(70.0407792639522,34.1567466380065,25.0000000000001));
#9214=CARTESIAN_POINT('Ctrl Pts',(71.0898199054102,33.4030260188376,25.0000000000001));
#9215=CARTESIAN_POINT('Ctrl Pts',(72.1402068924224,32.6581999429906,25.0000000000001));
#9216=CARTESIAN_POINT('Ctrl Pts',(72.3863913425034,32.4836313314639,25.0000000000001));
#9217=CARTESIAN_POINT('Ctrl Pts',(72.6326498509789,32.3095514218598,25.0000000000001));
#9218=CARTESIAN_POINT('Ctrl Pts',(72.8790059372784,32.1359538175003,25.0000000000001));
#9219=CARTESIAN_POINT('Ctrl Pts',(72.9286909378154,32.1009427195591,25.0000000000001));
#9220=CARTESIAN_POINT('Ctrl Pts',(72.9783799076115,32.0659512395566,25.0000000000001));
#9221=CARTESIAN_POINT('Ctrl Pts',(73.0280730400874,32.030979325534,25.0000000000001));
#9222=CARTESIAN_POINT('Ctrl Pts',(73.0635665772672,32.0060004830105,25.0000000000001));
#9223=CARTESIAN_POINT('Ctrl Pts',(73.0990697832648,31.9810263118437,25.0000000000001));
#9224=CARTESIAN_POINT('Ctrl Pts',(73.1345847051824,31.9560554193695,25.0000000000001));
#9225=CARTESIAN_POINT('Ctrl Pts',(74.1000277183134,31.2772428986274,25.0000000000001));
#9226=CARTESIAN_POINT('Ctrl Pts',(75.0736303041406,30.6012086898854,25.0000000000001));
#9227=CARTESIAN_POINT('Ctrl Pts',(76.0547670744571,29.9293290727267,25.0000000000001));
#9228=CARTESIAN_POINT('Ctrl Pts',(76.9745827966288,29.2994419316403,25.0000000000001));
#9229=CARTESIAN_POINT('Ctrl Pts',(77.9010206378247,28.6732065536317,25.0000000000001));
#9230=CARTESIAN_POINT('Ctrl Pts',(78.8335336207789,28.0517239817985,25.0000000000001));
#9231=CARTESIAN_POINT('Ctrl Pts',(79.7077645422984,27.4690840707048,25.0000000000001));
#9232=CARTESIAN_POINT('Ctrl Pts',(80.5873350480293,26.8906215256502,25.0000000000001));
#9233=CARTESIAN_POINT('Ctrl Pts',(81.4717631628992,26.3172112524276,25.0000000000001));
#9234=CARTESIAN_POINT('Ctrl Pts',(82.3009145205897,25.7796391212815,25.0000000000001));
#9235=CARTESIAN_POINT('Ctrl Pts',(83.1343352590044,25.2465074533943,25.0000000000001));
#9236=CARTESIAN_POINT('Ctrl Pts',(83.9715992196895,24.7185072927335,25.0000000000001));
#9237=CARTESIAN_POINT('Ctrl Pts',(84.3640667012607,24.4710072174237,25.0000000000001));
#9238=CARTESIAN_POINT('Ctrl Pts',(84.7573782112601,24.2246342293148,25.0000000000001));
#9239=CARTESIAN_POINT('Ctrl Pts',(85.151487452235,23.9794570370164,25.0000000000001));
#9240=CARTESIAN_POINT('Ctrl Pts',(85.2759172916967,23.9020486550107,25.0000000000001));
#9241=CARTESIAN_POINT('Ctrl Pts',(85.4004266383056,23.8247594596692,25.0000000000001));
#9242=CARTESIAN_POINT('Ctrl Pts',(85.5250140009801,23.7475915785448,25.0000000000001));
#9243=CARTESIAN_POINT('Ctrl Pts',(85.6006832213009,23.7007229935363,25.0000000000001));
#9244=CARTESIAN_POINT('Ctrl Pts',(85.6763761818179,23.6539022640716,25.0000000000001));
#9245=CARTESIAN_POINT('Ctrl Pts',(85.7521211486376,23.6071122170034,25.0000000000001));
#9246=CARTESIAN_POINT('Ctrl Pts',(86.8189992193685,22.9480680951102,25.0000000000001));
#9247=CARTESIAN_POINT('Ctrl Pts',(87.8953183319792,22.2956602946924,25.0000000000001));
#9248=CARTESIAN_POINT('Ctrl Pts',(88.9809339474695,21.6509533357167,25.0000000000001));
#9249=CARTESIAN_POINT('Ctrl Pts',(90.0187858805737,21.0346114610132,25.0000000000001));
#9250=CARTESIAN_POINT('Ctrl Pts',(91.0651344673981,20.4253078932095,25.0000000000001));
#9251=CARTESIAN_POINT('Ctrl Pts',(92.1198205279235,19.8239389045421,25.0000000000001));
#9252=CARTESIAN_POINT('Ctrl Pts',(93.1371001567188,19.2438986020696,25.0000000000001));
#9253=CARTESIAN_POINT('Ctrl Pts',(94.162136490687,18.6712401789023,25.0000000000001));
#9254=CARTESIAN_POINT('Ctrl Pts',(95.1947529130522,18.1067332667718,25.0000000000001));
#9255=CARTESIAN_POINT('Ctrl Pts',(96.196944163343,17.5588590747557,25.0000000000001));
#9256=CARTESIAN_POINT('Ctrl Pts',(97.2062755267639,17.0186632391373,25.0000000000001));
#9257=CARTESIAN_POINT('Ctrl Pts',(98.2225511036303,16.4868141437658,25.0000000000001));
#9258=CARTESIAN_POINT('Ctrl Pts',(98.4885714663643,16.3475972891142,25.0000000000001));
#9259=CARTESIAN_POINT('Ctrl Pts',(98.7550674415586,16.2089521416587,25.0000000000001));
#9260=CARTESIAN_POINT('Ctrl Pts',(99.0220350938054,16.0708902585445,25.0000000000001));
#9261=CARTESIAN_POINT('Ctrl Pts',(99.0971646665005,16.0320371233554,25.0000000000001));
#9262=CARTESIAN_POINT('Ctrl Pts',(99.1723388929282,15.9932264015618,25.0000000000001));
#9263=CARTESIAN_POINT('Ctrl Pts',(99.2475623772724,15.9544559749396,25.0000000000001));
#9264=CARTESIAN_POINT('Ctrl Pts',(100.299373993986,15.41234887286,25.0000000000001));
#9265=CARTESIAN_POINT('Ctrl Pts',(101.360529515776,14.8782723788936,25.0000000000001));
#9266=CARTESIAN_POINT('Ctrl Pts',(102.430907202419,14.3529815560378,25.0000000000001));
#9267=CARTESIAN_POINT('Ctrl Pts',(103.473274291026,13.8414370119714,25.0000000000001));
#9268=CARTESIAN_POINT('Ctrl Pts',(104.52438733127,13.3382244702285,25.0000000000001));
#9269=CARTESIAN_POINT('Ctrl Pts',(105.584100597309,12.8440072383845,25.0000000000001));
#9270=CARTESIAN_POINT('Ctrl Pts',(106.619814754682,12.360982442675,25.0000000000001));
#9271=CARTESIAN_POINT('Ctrl Pts',(107.663744132073,11.8865502575117,25.0000000000001));
#9272=CARTESIAN_POINT('Ctrl Pts',(108.715718557623,11.4212951390412,25.0000000000001));
#9273=CARTESIAN_POINT('Ctrl Pts',(109.74685733301,10.965254971666,25.0000000000001));
#9274=CARTESIAN_POINT('Ctrl Pts',(110.78572573032,10.5180320455846,25.0000000000001));
#9275=CARTESIAN_POINT('Ctrl Pts',(111.832128697192,10.0801413425618,25.0000000000001));
#9276=CARTESIAN_POINT('Ctrl Pts',(112.11045009164,9.96367153605378,25.0000000000001));
#9277=CARTESIAN_POINT('Ctrl Pts',(112.389304320048,9.8478617348605,25.0000000000001));
#9278=CARTESIAN_POINT('Ctrl Pts',(112.668687272398,9.73272118180913,25.0000000000001));
#9279=CARTESIAN_POINT('Ctrl Pts',(112.799648031312,9.6787490475663,25.0000000000001));
#9280=CARTESIAN_POINT('Ctrl Pts',(112.930724962206,9.62492396215648,25.0000000000001));
#9281=CARTESIAN_POINT('Ctrl Pts',(113.061917627266,9.57124686282096,25.0000000000001));
#9282=CARTESIAN_POINT('Ctrl Pts',(113.136076136524,9.54090512331734,25.0000000000001));
#9283=CARTESIAN_POINT('Ctrl Pts',(113.210271625404,9.51061066867802,25.0000000000001));
#9284=CARTESIAN_POINT('Ctrl Pts',(113.284504013508,9.4803636668373,25.0000000000001));
#9285=CARTESIAN_POINT('Ctrl Pts',(113.332364618527,9.4608622087127,25.0000000000001));
#9286=CARTESIAN_POINT('Ctrl Pts',(113.38023826595,9.44138140910595,25.0000000000001));
#9287=CARTESIAN_POINT('Ctrl Pts',(113.428132494267,9.4219182412191,25.0000000000001));
#9288=CARTESIAN_POINT('Ctrl Pts',(114.149202999218,9.12889094358361,25.0000000000001));
#9289=CARTESIAN_POINT('Ctrl Pts',(114.875975859862,8.83944349063256,25.0000000000001));
#9290=CARTESIAN_POINT('Ctrl Pts',(115.60777575188,8.55405656223017,25.0000000000001));
#9291=CARTESIAN_POINT('Ctrl Pts',(116.328331424398,8.27305464850276,25.0000000000001));
#9292=CARTESIAN_POINT('Ctrl Pts',(117.053760911735,7.99598951491613,25.0000000000001));
#9293=CARTESIAN_POINT('Ctrl Pts',(117.783384155275,7.72328397406765,25.0000000000001));
#9294=CARTESIAN_POINT('Ctrl Pts',(118.498966389033,7.45582643100485,25.0000000000001));
#9295=CARTESIAN_POINT('Ctrl Pts',(119.218582550737,7.19256232969555,25.0000000000001));
#9296=CARTESIAN_POINT('Ctrl Pts',(119.941556034713,6.9338548568966,25.0000000000001));
#9297=CARTESIAN_POINT('Ctrl Pts',(120.657883223477,6.67752568188564,25.0000000000001));
#9298=CARTESIAN_POINT('Ctrl Pts',(121.377506358092,6.42566980935821,25.0000000000001));
#9299=CARTESIAN_POINT('Ctrl Pts',(122.099731764364,6.1786043370424,25.0000000000001));
#9300=CARTESIAN_POINT('Ctrl Pts',(122.813510112138,5.93442851175294,25.0000000000001));
#9301=CARTESIAN_POINT('Ctrl Pts',(123.529830247605,5.69493171691093,25.0000000000001));
#9302=CARTESIAN_POINT('Ctrl Pts',(124.24798695059,5.46038386773084,25.0000000000001));
#9303=CARTESIAN_POINT('Ctrl Pts',(124.724609977416,5.30472020080811,25.0000000000001));
#9304=CARTESIAN_POINT('Ctrl Pts',(125.20204121732,5.15123562927839,25.0000000000001));
#9305=CARTESIAN_POINT('Ctrl Pts',(125.680065601264,5.,25.0000000000001));
#9306=CARTESIAN_POINT('Origin',(-85.4296283056384,23.8067054410608,-48.9999999999999));
#9307=CARTESIAN_POINT('',(-65.6680057154831,-5.,-48.9999999999999));
#9308=CARTESIAN_POINT('',(-20.,72.1122755947453,-48.9999999999999));
#9309=CARTESIAN_POINT('Ctrl Pts',(-37.,59.9327136539873,-48.9999999999999));
#9310=CARTESIAN_POINT('Ctrl Pts',(-63.6931530394793,38.6151528518972,-48.9999999999999));
#9311=CARTESIAN_POINT('Ctrl Pts',(-89.434492138698,16.4672437123984,-48.9999999999999));
#9312=CARTESIAN_POINT('Ctrl Pts',(-125.680065601287,4.99999999999283,-48.9999999999999));
#9313=CARTESIAN_POINT('Origin',(-85.4296283056384,23.8067054410608,-48.9999999999999));
#9314=CARTESIAN_POINT('',(20.,-5.,-48.9999999999999));
#9315=CARTESIAN_POINT('',(65.6680057154831,-5.,-48.9999999999999));
#9316=CARTESIAN_POINT('Ctrl Pts',(125.680065601293,4.99999999999088,-49.));
#9317=CARTESIAN_POINT('Ctrl Pts',(89.4344921387009,16.4672437123958,-49.));
#9318=CARTESIAN_POINT('Ctrl Pts',(63.6931530394808,38.615152851896,-48.9999999999999));
#9319=CARTESIAN_POINT('Ctrl Pts',(37.,59.9327136539873,-48.9999999999999));
#9320=CARTESIAN_POINT('Origin',(-145.859521458148,-5.,-58.9999999999999));
#9321=CARTESIAN_POINT('',(-145.859521458148,1.99649259469911E-14,-58.9999999999999));
#9322=CARTESIAN_POINT('Ctrl Pts',(-145.859521458148,2.04281036531029E-14,
-58.9999999999999));
#9323=CARTESIAN_POINT('Ctrl Pts',(-138.765903145325,1.29386700366004,-58.9999999999999));
#9324=CARTESIAN_POINT('Ctrl Pts',(-132.060245856665,2.9814615985512,-58.9999999999999));
#9325=CARTESIAN_POINT('Ctrl Pts',(-125.680065601889,4.99999999980248,-58.9999999999999));
#9326=CARTESIAN_POINT('',(-145.859521458148,1.99493199737333E-14,-58.9999999999999));
#9327=CARTESIAN_POINT('Origin',(-145.859521458148,-5.,-58.9999999999999));
#9328=CARTESIAN_POINT('',(145.859521458148,1.99493199737333E-14,-59.));
#9329=CARTESIAN_POINT('',(145.859521458148,1.99493199737333E-14,-59.));
#9330=CARTESIAN_POINT('Ctrl Pts',(145.859521458148,1.99966320462804E-14,
-59.));
#9331=CARTESIAN_POINT('Ctrl Pts',(139.935495507955,1.08053483677362,-59.));
#9332=CARTESIAN_POINT('Ctrl Pts',(134.282043748658,2.43566561952013,-59.));
#9333=CARTESIAN_POINT('Ctrl Pts',(127.792835858247,4.34336551753063,-59.));
#9334=CARTESIAN_POINT('Ctrl Pts',(126.732026641956,4.6671843627512,-59.));
#9335=CARTESIAN_POINT('Ctrl Pts',(125.68006560189,4.99999999980207,-59.));
#9336=CARTESIAN_POINT('Origin',(-145.859521458148,-5.,144.542028553823));
#9337=CARTESIAN_POINT('',(-145.859521458148,0.,35.0000000000001));
#9338=CARTESIAN_POINT('',(-36.8276756314269,0.,133.982075177761));
#9339=CARTESIAN_POINT('Ctrl Pts',(-145.859521458148,8.23993651088983E-17,
35.0000000000001));
#9340=CARTESIAN_POINT('Ctrl Pts',(-145.635702363577,0.000231282962457004,
35.0000000000001));
#9341=CARTESIAN_POINT('Ctrl Pts',(-145.411883255014,0.000447783512624677,
35.0006859694096));
#9342=CARTESIAN_POINT('Ctrl Pts',(-145.188067286082,0.000650024992512574,
35.0020579084857));
#9343=CARTESIAN_POINT('Ctrl Pts',(-139.052999252432,0.00619371004421888,
35.0396644278488));
#9344=CARTESIAN_POINT('Ctrl Pts',(-132.962545444182,-5.00267456489816E-15,
35.5922856589093));
#9345=CARTESIAN_POINT('Ctrl Pts',(-126.977116946521,5.75982404132925E-15,
36.6397078209221));
#9346=CARTESIAN_POINT('Ctrl Pts',(-123.729336577937,-8.83548270628736E-15,
37.2080542871332));
#9347=CARTESIAN_POINT('Ctrl Pts',(-120.512481495569,6.22417271669332E-15,
37.9221153240664));
#9348=CARTESIAN_POINT('Ctrl Pts',(-117.336234309904,2.03055396797011E-14,
38.7787168150856));
#9349=CARTESIAN_POINT('Ctrl Pts',(-114.085205078277,2.1960099348902E-14,
39.6554862616599));
#9350=CARTESIAN_POINT('Ctrl Pts',(-110.876720955834,-3.26284544765647E-14,
40.6815897913547));
#9351=CARTESIAN_POINT('Ctrl Pts',(-107.721164151354,-1.36321397827812E-14,
41.8535592808524));
#9352=CARTESIAN_POINT('Ctrl Pts',(-104.5107545404,-2.00540520775008E-14,
43.0459010277944));
#9353=CARTESIAN_POINT('Ctrl Pts',(-101.355129960869,-4.96859830016179E-14,
44.3892216824941));
#9354=CARTESIAN_POINT('Ctrl Pts',(-98.2651875381795,-8.7145968338722E-15,
45.8797997202868));
#9355=CARTESIAN_POINT('Ctrl Pts',(-95.1416080119443,2.68306712685109E-14,
47.3866041859354));
#9356=CARTESIAN_POINT('Ctrl Pts',(-92.0851458120305,-2.46012083690602E-14,
49.0438828741843));
#9357=CARTESIAN_POINT('Ctrl Pts',(-89.1070253835134,-4.47091941648079E-15,
50.8477906894533));
#9358=CARTESIAN_POINT('Ctrl Pts',(-86.116852734007,1.31897776828331E-14,
52.6589987788904));
#9359=CARTESIAN_POINT('Ctrl Pts',(-83.2056472832304,-2.52433361746903E-14,
54.6180166790272));
#9360=CARTESIAN_POINT('Ctrl Pts',(-80.384830163582,-3.25227617460708E-14,
56.7210696683281));
#9361=CARTESIAN_POINT('Ctrl Pts',(-77.5611534148143,-5.45739529723217E-14,
58.8262546468053));
#9362=CARTESIAN_POINT('Ctrl Pts',(-74.838114010143,-1.58426147313227E-14,
61.0685191399763));
#9363=CARTESIAN_POINT('Ctrl Pts',(-72.2297132774974,-3.95963338885915E-14,
63.4364962704633));
#9364=CARTESIAN_POINT('Ctrl Pts',(-69.6213194790221,-7.79039001579624E-14,
65.8044671059218));
#9365=CARTESIAN_POINT('Ctrl Pts',(-67.1275347240086,-6.25228860961752E-14,
68.2980716005042));
#9366=CARTESIAN_POINT('Ctrl Pts',(-64.7594023581045,-8.88178419700125E-14,
70.9062580231546));
#9367=CARTESIAN_POINT('Ctrl Pts',(-62.4021012990926,-9.12248625477642E-14,
73.5025151854382));
#9368=CARTESIAN_POINT('Ctrl Pts',(-60.169846560561,-4.0610067571623E-14,
76.2117317741152));
#9369=CARTESIAN_POINT('Ctrl Pts',(-58.0726499521868,-6.27156238454472E-14,
79.0216408040367));
#9370=CARTESIAN_POINT('Ctrl Pts',(-55.9948328500291,-7.60233291321462E-14,
81.8055843859426));
#9371=CARTESIAN_POINT('Ctrl Pts',(-54.0490749518655,-1.67744203884114E-13,
84.6891394721334));
#9372=CARTESIAN_POINT('Ctrl Pts',(-52.2449416359332,-1.38934194302791E-13,
87.6582306461879));
#9373=CARTESIAN_POINT('Ctrl Pts',(-50.4652489916243,-1.05237142154808E-13,
90.5870994144124));
#9374=CARTESIAN_POINT('Ctrl Pts',(-48.8232383526347,-1.1932076725731E-13,
93.5993053079782));
#9375=CARTESIAN_POINT('Ctrl Pts',(-47.3258881353928,-1.2706433568353E-13,
96.6820335276708));
#9376=CARTESIAN_POINT('Ctrl Pts',(-45.855086603224,-1.35827824389417E-13,
99.7101036054481));
#9377=CARTESIAN_POINT('Ctrl Pts',(-44.5237168473912,-7.3722747694714E-14,
102.806759783349));
#9378=CARTESIAN_POINT('Ctrl Pts',(-43.3384647873198,-7.32425154326057E-14,
105.955904638828));
#9379=CARTESIAN_POINT('Ctrl Pts',(-42.1784113697529,-6.02896671181379E-14,
109.038098186581));
#9380=CARTESIAN_POINT('Ctrl Pts',(-41.1578799651057,-1.27995749366182E-13,
112.171204882295));
#9381=CARTESIAN_POINT('Ctrl Pts',(-40.2800279987792,-1.24975527024613E-13,
115.345683225176));
#9382=CARTESIAN_POINT('Ctrl Pts',(-38.5944013814798,-1.62104376724653E-13,
121.441227116469));
#9383=CARTESIAN_POINT('Ctrl Pts',(-37.4373840532588,-5.41978339669594E-15,
127.68681682945));
#9384=CARTESIAN_POINT('Ctrl Pts',(-36.8276756314269,-1.16656359051837E-13,
133.982075177761));
#9385=CARTESIAN_POINT('',(-145.859521458148,-5.,35.0000000000001));
#9386=CARTESIAN_POINT('',(-36.8276756314269,-5.,133.982075177761));
#9387=CARTESIAN_POINT('Origin',(145.859521458148,-5.,144.542028553823));
#9388=CARTESIAN_POINT('',(145.859521458148,6.34121985785824E-17,35.0000000000001));
#9389=CARTESIAN_POINT('',(36.827675631427,0.,133.982075177761));
#9390=CARTESIAN_POINT('Ctrl Pts',(145.859521458148,3.17060992892912E-17,
35.0000000000001));
#9391=CARTESIAN_POINT('Ctrl Pts',(145.635702363633,0.000231282959717141,
35.0000000000001));
#9392=CARTESIAN_POINT('Ctrl Pts',(145.41188325512,0.000447783510709151,
35.0006859694093));
#9393=CARTESIAN_POINT('Ctrl Pts',(145.18806728624,0.00065002499126718,35.0020579084847));
#9394=CARTESIAN_POINT('Ctrl Pts',(139.052999252553,0.00619371003938468,
35.0396644278391));
#9395=CARTESIAN_POINT('Ctrl Pts',(132.962545444248,2.81306248191126E-14,
35.5922856588977));
#9396=CARTESIAN_POINT('Ctrl Pts',(126.977116946521,-1.25959050860987E-14,
36.6397078209221));
#9397=CARTESIAN_POINT('Ctrl Pts',(123.729336577941,-1.22807761130853E-14,
37.2080542871325));
#9398=CARTESIAN_POINT('Ctrl Pts',(120.512481495573,-2.84858070297575E-14,
37.9221153240654));
#9399=CARTESIAN_POINT('Ctrl Pts',(117.336234309904,1.86685976871553E-14,
38.7787168150856));
#9400=CARTESIAN_POINT('Ctrl Pts',(114.08520507828,4.21595021817856E-14,
39.6554862616589));
#9401=CARTESIAN_POINT('Ctrl Pts',(110.876720955837,-1.07034139801461E-15,
40.6815897913534));
#9402=CARTESIAN_POINT('Ctrl Pts',(107.721164151354,-3.37470208163848E-14,
41.8535592808524));
#9403=CARTESIAN_POINT('Ctrl Pts',(104.510754540403,-4.76367518704849E-14,
43.0459010277931));
#9404=CARTESIAN_POINT('Ctrl Pts',(101.355129960872,-3.43757017307364E-14,
44.3892216824924));
#9405=CARTESIAN_POINT('Ctrl Pts',(98.2651875381796,-2.63709732083997E-14,
45.8797997202868));
#9406=CARTESIAN_POINT('Ctrl Pts',(95.1416080119479,1.09021272333422E-14,
47.3866041859337));
#9407=CARTESIAN_POINT('Ctrl Pts',(92.0851458120341,1.05042416094065E-16,
49.0438828741821));
#9408=CARTESIAN_POINT('Ctrl Pts',(89.1070253835135,3.41156072033826E-15,
50.8477906894532));
#9409=CARTESIAN_POINT('Ctrl Pts',(86.1168527340107,1.03272048229725E-14,
52.6589987788881));
#9410=CARTESIAN_POINT('Ctrl Pts',(83.2056472832341,5.36384240903567E-14,
54.6180166790245));
#9411=CARTESIAN_POINT('Ctrl Pts',(80.3848301635821,3.08073424156598E-14,
56.721069668328));
#9412=CARTESIAN_POINT('Ctrl Pts',(77.5611534148135,1.32010255714472E-14,
58.8262546468059));
#9413=CARTESIAN_POINT('Ctrl Pts',(74.8381140101423,1.51039607992001E-14,
61.068519139977));
#9414=CARTESIAN_POINT('Ctrl Pts',(72.2297132774974,2.42097771138098E-14,
63.4364962704633));
#9415=CARTESIAN_POINT('Ctrl Pts',(69.6213194790238,1.66550167885819E-14,
65.8044671059204));
#9416=CARTESIAN_POINT('Ctrl Pts',(67.1275347240088,4.55894098149439E-14,
68.298071600504));
#9417=CARTESIAN_POINT('Ctrl Pts',(64.7594023581046,1.11217543556858E-14,
70.9062580231545));
#9418=CARTESIAN_POINT('Ctrl Pts',(62.4021012990924,-1.57438813545332E-14,
73.5025151854384));
#9419=CARTESIAN_POINT('Ctrl Pts',(60.1698465605612,-5.22446090150672E-14,
76.211731774115));
#9420=CARTESIAN_POINT('Ctrl Pts',(58.0726499521868,-2.90860017955518E-14,
79.0216408040366));
#9421=CARTESIAN_POINT('Ctrl Pts',(55.9948328500282,3.31444783804878E-15,
81.8055843859439));
#9422=CARTESIAN_POINT('Ctrl Pts',(54.0490749518631,-4.6343826823798E-14,
84.6891394721373));
#9423=CARTESIAN_POINT('Ctrl Pts',(52.2449416359332,-3.83898540398404E-14,
87.6582306461879));
#9424=CARTESIAN_POINT('Ctrl Pts',(50.4652489916249,-5.26518919980718E-14,
90.5870994144115));
#9425=CARTESIAN_POINT('Ctrl Pts',(48.8232383526351,1.12664867902641E-14,
93.5993053079775));
#9426=CARTESIAN_POINT('Ctrl Pts',(47.3258881353929,2.19975239907418E-14,
96.6820335276706));
#9427=CARTESIAN_POINT('Ctrl Pts',(45.8550866032248,3.66910777152371E-14,
99.7101036054466));
#9428=CARTESIAN_POINT('Ctrl Pts',(44.5237168473917,-5.11013660504775E-14,
102.806759783348));
#9429=CARTESIAN_POINT('Ctrl Pts',(43.3384647873199,-9.3811914345706E-14,
105.955904638828));
#9430=CARTESIAN_POINT('Ctrl Pts',(42.178411369753,-1.41776291118567E-13,
109.038098186581));
#9431=CARTESIAN_POINT('Ctrl Pts',(41.1578799651058,-8.19907887432609E-14,
112.171204882295));
#9432=CARTESIAN_POINT('Ctrl Pts',(40.2800279987793,-4.11497414918791E-14,
115.345683225176));
#9433=CARTESIAN_POINT('Ctrl Pts',(38.5944013814794,5.4727582458512E-14,
121.44122711647));
#9434=CARTESIAN_POINT('Ctrl Pts',(37.4373840532589,1.27133044339828E-13,
127.686816829449));
#9435=CARTESIAN_POINT('Ctrl Pts',(36.827675631427,-8.1444996146568E-14,
133.982075177761));
#9436=CARTESIAN_POINT('',(36.827675631427,-5.,133.982075177761));
#9437=CARTESIAN_POINT('',(145.859521458148,-5.,35.0000000000001));
#9438=CARTESIAN_POINT('Origin',(0.,-5.,130.415240784856));
#9439=CARTESIAN_POINT('Ctrl Pts',(-36.8276756314269,0.,133.982075177761));
#9440=CARTESIAN_POINT('Ctrl Pts',(-36.6797497079439,0.,135.50941492147));
#9441=CARTESIAN_POINT('Ctrl Pts',(-36.4288634825457,0.,137.114741394618));
#9442=CARTESIAN_POINT('Ctrl Pts',(-36.0405708212051,0.,138.786456639301));
#9443=CARTESIAN_POINT('Ctrl Pts',(-35.6522781598644,0.,140.458171883983));
#9444=CARTESIAN_POINT('Ctrl Pts',(-35.126304365244,0.,142.196602013066));
#9445=CARTESIAN_POINT('Ctrl Pts',(-34.4253505833173,0.,143.976038593824));
#9446=CARTESIAN_POINT('Ctrl Pts',(-33.7243968013906,0.,145.755475174581));
#9447=CARTESIAN_POINT('Ctrl Pts',(-32.8479279009936,0.,147.576162799206));
#9448=CARTESIAN_POINT('Ctrl Pts',(-31.7618111665595,0.,149.393843247098));
#9449=CARTESIAN_POINT('Ctrl Pts',(-30.6756944321254,0.,151.21152369499));
#9450=CARTESIAN_POINT('Ctrl Pts',(-29.3791356772816,0.,153.026147945389));
#9451=CARTESIAN_POINT('Ctrl Pts',(-27.8512109316029,0.,154.773197383129));
#9452=CARTESIAN_POINT('Ctrl Pts',(-26.3232861859242,0.,156.52024682087));
#9453=CARTESIAN_POINT('Ctrl Pts',(-24.5631346628349,0.,158.199131371192));
#9454=CARTESIAN_POINT('Ctrl Pts',(-22.5757614892594,0.,159.729656917198));
#9455=CARTESIAN_POINT('Ctrl Pts',(-20.5883883156839,0.,161.260182463203));
#9456=CARTESIAN_POINT('Ctrl Pts',(-18.3733019437227,0.,162.641132549651));
#9457=CARTESIAN_POINT('Ctrl Pts',(-15.972090553586,0.,163.790266228263));
#9458=CARTESIAN_POINT('Ctrl Pts',(-13.5708791634494,0.,164.939399906875));
#9459=CARTESIAN_POINT('Ctrl Pts',(-10.9839174320016,0.,165.855200551742));
#9460=CARTESIAN_POINT('Ctrl Pts',(-8.29064013714808,0.,166.474432208352));
#9461=CARTESIAN_POINT('Ctrl Pts',(-5.59736284229456,0.,167.093663864962));
#9462=CARTESIAN_POINT('Ctrl Pts',(-2.79913386299196,0.,167.415240784856));
#9463=CARTESIAN_POINT('Ctrl Pts',(1.41553435639707E-14,0.,167.415240784856));
#9464=CARTESIAN_POINT('Ctrl Pts',(2.79913386299198,0.,167.415240784856));
#9465=CARTESIAN_POINT('Ctrl Pts',(5.59736284229459,0.,167.093663864962));
#9466=CARTESIAN_POINT('Ctrl Pts',(8.29064013714809,0.,166.474432208352));
#9467=CARTESIAN_POINT('Ctrl Pts',(10.9839174320016,0.,165.855200551742));
#9468=CARTESIAN_POINT('Ctrl Pts',(13.5708791634494,0.,164.939399906875));
#9469=CARTESIAN_POINT('Ctrl Pts',(15.9720905535861,0.,163.790266228263));
#9470=CARTESIAN_POINT('Ctrl Pts',(18.3733019437227,0.,162.641132549651));
#9471=CARTESIAN_POINT('Ctrl Pts',(20.588388315684,0.,161.260182463203));
#9472=CARTESIAN_POINT('Ctrl Pts',(22.5757614892594,0.,159.729656917197));
#9473=CARTESIAN_POINT('Ctrl Pts',(24.5631346628349,0.,158.199131371192));
#9474=CARTESIAN_POINT('Ctrl Pts',(26.3232861859243,0.,156.52024682087));
#9475=CARTESIAN_POINT('Ctrl Pts',(27.851210931603,0.,154.773197383129));
#9476=CARTESIAN_POINT('Ctrl Pts',(29.3791356772816,0.,153.026147945389));
#9477=CARTESIAN_POINT('Ctrl Pts',(30.6756944321254,0.,151.21152369499));
#9478=CARTESIAN_POINT('Ctrl Pts',(31.7618111665595,0.,149.393843247098));
#9479=CARTESIAN_POINT('Ctrl Pts',(32.8479279009937,0.,147.576162799206));
#9480=CARTESIAN_POINT('Ctrl Pts',(33.7243968013906,0.,145.755475174581));
#9481=CARTESIAN_POINT('Ctrl Pts',(34.4253505833173,0.,143.976038593824));
#9482=CARTESIAN_POINT('Ctrl Pts',(35.126304365244,0.,142.196602013066));
#9483=CARTESIAN_POINT('Ctrl Pts',(35.6522781598644,0.,140.458171883983));
#9484=CARTESIAN_POINT('Ctrl Pts',(36.0405708212051,0.,138.786456639301));
#9485=CARTESIAN_POINT('Ctrl Pts',(36.4288634825457,0.,137.114741394618));
#9486=CARTESIAN_POINT('Ctrl Pts',(36.6797497079439,0.,135.50941492147));
#9487=CARTESIAN_POINT('Ctrl Pts',(36.8276756314269,0.,133.982075177761));
#9488=CARTESIAN_POINT('Ctrl Pts',(145.859521458148,3.17060992892912E-17,
35.0000000000001));
#9489=CARTESIAN_POINT('Ctrl Pts',(145.859521458148,3.17060992892912E-17,
35.0000000000001));
#9490=CARTESIAN_POINT('Ctrl Pts',(139.935495507955,1.0805348367736,35.0000000000001));
#9491=CARTESIAN_POINT('Ctrl Pts',(139.721849114783,-0.00946396649206172,
35.0000000000001));
#9492=CARTESIAN_POINT('Ctrl Pts',(134.282043748658,2.43566561952011,35.0000000000001));
#9493=CARTESIAN_POINT('Ctrl Pts',(133.377109515712,-0.02133300752971,35.5229040509096));
#9494=CARTESIAN_POINT('Ctrl Pts',(126.153138109028,4.82540450931202,35.0000000000001));
#9495=CARTESIAN_POINT('Ctrl Pts',(123.752347112548,-0.0422637614564399,
37.2196520098122));
#9496=CARTESIAN_POINT('Ctrl Pts',(123.502048229037,5.68149125852134,35.0000000000001));
#9497=CARTESIAN_POINT('Ctrl Pts',(120.526890370995,-0.0497618781603927,
37.9367613539355));
#9498=CARTESIAN_POINT('Ctrl Pts',(118.307860920989,7.50353712828282,35.0000000000001));
#9499=CARTESIAN_POINT('Ctrl Pts',(114.083064301351,-0.0657204391170305,
39.6868647729585));
#9500=CARTESIAN_POINT('Ctrl Pts',(115.764763492932,8.46949624883498,35.0000000000001));
#9501=CARTESIAN_POINT('Ctrl Pts',(110.864745388532,-0.0741808833697154,
40.7198997814395));
#9502=CARTESIAN_POINT('Ctrl Pts',(110.777462874248,10.5021449940676,35.0000000000001));
#9503=CARTESIAN_POINT('Ctrl Pts',(104.480363407898,-0.091984029515797,43.1072738736836));
#9504=CARTESIAN_POINT('Ctrl Pts',(108.33325968362,11.568834618748,35.0000000000001));
#9505=CARTESIAN_POINT('Ctrl Pts',(101.314363685346,-0.101326731409194,44.4616401695737));
#9506=CARTESIAN_POINT('Ctrl Pts',(103.53464932529,13.7938025050227,35.0000000000001));
#9507=CARTESIAN_POINT('Ctrl Pts',(95.0816761504739,-0.120814322928678,47.488542779257));
#9508=CARTESIAN_POINT('Ctrl Pts',(101.180242157587,14.9520807666169,35.0000000000001));
#9509=CARTESIAN_POINT('Ctrl Pts',(92.0150600641061,-0.130959212554766,49.1610880733554));
#9510=CARTESIAN_POINT('Ctrl Pts',(96.5521256306011,17.3510840595046,35.0000000000001));
#9511=CARTESIAN_POINT('Ctrl Pts',(86.0280376785636,-0.151971109631613,52.8121020506907));
#9512=CARTESIAN_POINT('Ctrl Pts',(94.2784162713182,18.591809090798,35.0000000000001));
#9513=CARTESIAN_POINT('Ctrl Pts',(83.1077052252586,-0.162838117082372,54.790558780279));
#9514=CARTESIAN_POINT('Ctrl Pts',(89.8025971466679,21.1465640558695,35.0000000000001));
#9515=CARTESIAN_POINT('Ctrl Pts',(77.4577804126425,-0.18521417990054,59.0320726395877));
#9516=CARTESIAN_POINT('Ctrl Pts',(87.6004873813004,22.4605939896476,35.0000000000001));
#9517=CARTESIAN_POINT('Ctrl Pts',(74.7282568878096,-0.19672323526795,61.2950966764346));
#9518=CARTESIAN_POINT('Ctrl Pts',(83.2587692299763,25.1528168924739,35.0000000000001));
#9519=CARTESIAN_POINT('Ctrl Pts',(69.4999442605203,-0.220303324011399,66.0760233448773));
#9520=CARTESIAN_POINT('Ctrl Pts',(81.1191608440196,26.5310098615222,35.0000000000001));
#9521=CARTESIAN_POINT('Ctrl Pts',(67.0012121018892,-0.232374357387438,68.5938742813195));
#9522=CARTESIAN_POINT('Ctrl Pts',(76.8933472370124,29.3424169676742,35.0000000000001));
#9523=CARTESIAN_POINT('Ctrl Pts',(62.2680278203847,-0.256998332240127,73.8476184739701));
#9524=CARTESIAN_POINT('Ctrl Pts',(74.8071420159619,30.7756311047781,35.0000000000001));
#9525=CARTESIAN_POINT('Ctrl Pts',(60.0336152719651,-0.269551273716776,76.583446406475));
#9526=CARTESIAN_POINT('Ctrl Pts',(70.6790365242624,33.6879386798268,35.0000000000001));
#9527=CARTESIAN_POINT('Ctrl Pts',(55.8546997737931,-0.295058994862664,82.2309706047639));
#9528=CARTESIAN_POINT('Ctrl Pts',(68.6371362536135,35.1670321177717,35.0000000000001));
#9529=CARTESIAN_POINT('Ctrl Pts',(53.9102158408265,-0.308013774531903,85.1425945209522));
#9530=CARTESIAN_POINT('Ctrl Pts',(64.5885424482125,38.1619564272879,35.0000000000001));
#9531=CARTESIAN_POINT('Ctrl Pts',(50.3279822508715,-0.334245102154949,91.0962909513875));
#9532=CARTESIAN_POINT('Ctrl Pts',(62.5818489134604,39.6777872988593,35.0000000000001));
#9533=CARTESIAN_POINT('Ctrl Pts',(48.6902305698515,-0.347521650108757,94.1382912080291));
#9534=CARTESIAN_POINT('Ctrl Pts',(58.5945703653485,42.7370446084141,35.0000000000001));
#9535=CARTESIAN_POINT('Ctrl Pts',(45.729227108235,-0.374316444392921,100.306271688078));
#9536=CARTESIAN_POINT('Ctrl Pts',(56.6139853519887,44.2804710463974,35.0000000000001));
#9537=CARTESIAN_POINT('Ctrl Pts',(44.4059543487921,-0.387834690723277,103.432186237973));
#9538=CARTESIAN_POINT('Ctrl Pts',(52.6698256321568,47.3857776215616,35.0000000000001));
#9539=CARTESIAN_POINT('Ctrl Pts',(42.0729707183869,-0.415032811852518,109.722571033699));
#9540=CARTESIAN_POINT('Ctrl Pts',(50.7062509256847,48.9476577587424,35.0000000000001));
#9541=CARTESIAN_POINT('Ctrl Pts',(41.063223964567,-0.428712686651402,112.886987153028));
#9542=CARTESIAN_POINT('Ctrl Pts',(44.8273949448428,53.6472659182591,35.0000000000001));
#9543=CARTESIAN_POINT('Ctrl Pts',(38.4911694061933,-0.469874648888817,122.374221150099));
#9544=CARTESIAN_POINT('Ctrl Pts',(40.9239818090477,56.7989616885694,35.0000000000001));
#9545=CARTESIAN_POINT('Ctrl Pts',(37.3884769379574,-0.497479074168109,128.688287898515));
#9546=CARTESIAN_POINT('Ctrl Pts',(37.,59.9327136539873,35.0000000000001));
#9547=CARTESIAN_POINT('Ctrl Pts',(36.826166312158,-0.524926336936336,134.849019038261));
#9548=CARTESIAN_POINT('',(37.,59.9327136539873,35.0000000000001));
#9549=CARTESIAN_POINT('Ctrl Pts',(37.,59.9327136539873,35.0000000000001));
#9550=CARTESIAN_POINT('Ctrl Pts',(63.6931530394734,38.6151528519019,35.0000000000001));
#9551=CARTESIAN_POINT('Ctrl Pts',(89.4344921386865,16.4672437124081,35.0000000000001));
#9552=CARTESIAN_POINT('Ctrl Pts',(125.680065601263,5.0000000000004,35.0000000000001));
#9553=CARTESIAN_POINT('',(37.,59.9327136539873,35.0000000000001));
#9554=CARTESIAN_POINT('Ctrl Pts',(145.859521458148,3.17060992892912E-17,
35.0000000000001));
#9555=CARTESIAN_POINT('Ctrl Pts',(139.935495507955,1.0805348367736,35.0000000000001));
#9556=CARTESIAN_POINT('Ctrl Pts',(134.282043748658,2.43566561952011,35.0000000000001));
#9557=CARTESIAN_POINT('Ctrl Pts',(127.792835858035,4.34336551759297,35.0000000000001));
#9558=CARTESIAN_POINT('Ctrl Pts',(126.732026641535,4.66718436287958,35.0000000000001));
#9559=CARTESIAN_POINT('Ctrl Pts',(125.680065601264,5.,35.0000000000001));
#9560=CARTESIAN_POINT('Ctrl Pts',(-37.,59.9327136539873,35.0000000000001));
#9561=CARTESIAN_POINT('Ctrl Pts',(-36.8261663120238,-0.524926383580335,
134.849019115296));
#9562=CARTESIAN_POINT('Ctrl Pts',(-40.9239818090476,56.7989616885694,35.0000000000001));
#9563=CARTESIAN_POINT('Ctrl Pts',(-37.3884769352297,-0.497479118373195,
128.688287970797));
#9564=CARTESIAN_POINT('Ctrl Pts',(-44.8273949448428,53.6472659182591,35.0000000000001));
#9565=CARTESIAN_POINT('Ctrl Pts',(-38.4911694013047,-0.469874690641024,
122.374221217509));
#9566=CARTESIAN_POINT('Ctrl Pts',(-50.7062509256847,48.9476577587424,35.0000000000001));
#9567=CARTESIAN_POINT('Ctrl Pts',(-41.0632239571272,-0.428712724746032,
112.886987213119));
#9568=CARTESIAN_POINT('Ctrl Pts',(-52.6698256321568,47.3857776215616,35.0000000000001));
#9569=CARTESIAN_POINT('Ctrl Pts',(-42.0729707102112,-0.415032848731579,
109.722571091349));
#9570=CARTESIAN_POINT('Ctrl Pts',(-56.6139853519887,44.2804710463974,35.0000000000001));
#9571=CARTESIAN_POINT('Ctrl Pts',(-44.4059543393734,-0.387834725185562,
103.432186290769));
#9572=CARTESIAN_POINT('Ctrl Pts',(-58.5945703653485,42.7370446084141,35.0000000000001));
#9573=CARTESIAN_POINT('Ctrl Pts',(-45.7292270983091,-0.374316477654,100.306271738463));
#9574=CARTESIAN_POINT('Ctrl Pts',(-62.5818489134604,39.6777872988593,35.0000000000001));
#9575=CARTESIAN_POINT('Ctrl Pts',(-48.6902305591338,-0.347521680988899,
94.1382912536552));
#9576=CARTESIAN_POINT('Ctrl Pts',(-64.5885424482124,38.1619564272879,35.0000000000001));
#9577=CARTESIAN_POINT('Ctrl Pts',(-50.3279822398692,-0.334245131855361,
91.0962909946666));
#9578=CARTESIAN_POINT('Ctrl Pts',(-68.6371362536135,35.1670321177717,35.0000000000001));
#9579=CARTESIAN_POINT('Ctrl Pts',(-53.9102158294643,-0.308013801901447,
85.1425945596379));
#9580=CARTESIAN_POINT('Ctrl Pts',(-70.6790365242624,33.6879386798268,35.0000000000001));
#9581=CARTESIAN_POINT('Ctrl Pts',(-55.8546997623558,-0.29505902108107,82.2309706412034));
#9582=CARTESIAN_POINT('Ctrl Pts',(-74.8071420159619,30.7756311047781,35.0000000000001));
#9583=CARTESIAN_POINT('Ctrl Pts',(-60.033615260567,-0.269551297668613,76.5834464385573));
#9584=CARTESIAN_POINT('Ctrl Pts',(-76.8933472370124,29.3424169676743,35.0000000000001));
#9585=CARTESIAN_POINT('Ctrl Pts',(-62.2680278091009,-0.256998355076532,
73.8476185039417));
#9586=CARTESIAN_POINT('Ctrl Pts',(-81.1191608440196,26.5310098615222,35.0000000000001));
#9587=CARTESIAN_POINT('Ctrl Pts',(-67.0012120909969,-0.232374378035801,
68.5938743072377));
#9588=CARTESIAN_POINT('Ctrl Pts',(-83.2587692299763,25.152816892474,35.0000000000001));
#9589=CARTESIAN_POINT('Ctrl Pts',(-69.499944249905,-0.220303343587152,66.0760233688529));
#9590=CARTESIAN_POINT('Ctrl Pts',(-87.6004873813004,22.4605939896476,35.0000000000001));
#9591=CARTESIAN_POINT('Ctrl Pts',(-74.7282568778784,-0.196723252748419,
61.2950966967217));
#9592=CARTESIAN_POINT('Ctrl Pts',(-89.8025971466678,21.1465640558695,35.0000000000001));
#9593=CARTESIAN_POINT('Ctrl Pts',(-77.4577804031182,-0.185214196358336,
59.0320726581288));
#9594=CARTESIAN_POINT('Ctrl Pts',(-94.2784162713182,18.591809090798,35.0000000000001));
#9595=CARTESIAN_POINT('Ctrl Pts',(-83.1077052166401,-0.162838131551871,
54.7905587955477));
#9596=CARTESIAN_POINT('Ctrl Pts',(-96.5521256306011,17.3510840595046,35.0000000000001));
#9597=CARTESIAN_POINT('Ctrl Pts',(-86.0280376704441,-0.15197112313549,52.812102064433));
#9598=CARTESIAN_POINT('Ctrl Pts',(-101.180242157587,14.9520807666169,35.0000000000001));
#9599=CARTESIAN_POINT('Ctrl Pts',(-92.0150600570349,-0.130959224191564,
49.1610880842809));
#9600=CARTESIAN_POINT('Ctrl Pts',(-103.53464932529,13.7938025050227,35.0000000000001));
#9601=CARTESIAN_POINT('Ctrl Pts',(-95.0816761439523,-0.120814333664019,
47.4885427888921));
#9602=CARTESIAN_POINT('Ctrl Pts',(-108.33325968362,11.568834618748,35.0000000000001));
#9603=CARTESIAN_POINT('Ctrl Pts',(-101.314363679931,-0.101326740412903,
44.4616401768735));
#9604=CARTESIAN_POINT('Ctrl Pts',(-110.777462874248,10.5021449940676,35.0000000000001));
#9605=CARTESIAN_POINT('Ctrl Pts',(-104.48036340304,-0.0919840376893306,
43.1072738799385));
#9606=CARTESIAN_POINT('Ctrl Pts',(-115.764763492932,8.46949624883498,35.0000000000001));
#9607=CARTESIAN_POINT('Ctrl Pts',(-110.864745384751,-0.0741808899612938,
40.7198997858525));
#9608=CARTESIAN_POINT('Ctrl Pts',(-118.307860920989,7.50353712828282,35.0000000000001));
#9609=CARTESIAN_POINT('Ctrl Pts',(-114.083064298091,-0.0657204449568292,
39.6868647765745));
#9610=CARTESIAN_POINT('Ctrl Pts',(-123.502048229037,5.68149125852133,35.0000000000001));
#9611=CARTESIAN_POINT('Ctrl Pts',(-120.5268903687,-0.0497618825821426,37.9367613562013));
#9612=CARTESIAN_POINT('Ctrl Pts',(-126.153138109028,4.82540450931201,35.0000000000001));
#9613=CARTESIAN_POINT('Ctrl Pts',(-123.752347110696,-0.0422637652119208,
37.2196520115247));
#9614=CARTESIAN_POINT('Ctrl Pts',(-134.282043748658,2.43566561952011,35.0000000000001));
#9615=CARTESIAN_POINT('Ctrl Pts',(-133.377109515013,-0.0213330094253222,
35.5229040513131));
#9616=CARTESIAN_POINT('Ctrl Pts',(-139.935495507955,1.08053483677359,35.0000000000001));
#9617=CARTESIAN_POINT('Ctrl Pts',(-139.721849114618,-0.00946396733301255,
35.0000000000001));
#9618=CARTESIAN_POINT('Ctrl Pts',(-145.859521458148,3.17060992892922E-17,
35.0000000000001));
#9619=CARTESIAN_POINT('Ctrl Pts',(-145.859521458148,3.17060992892922E-17,
35.0000000000001));
#9620=CARTESIAN_POINT('Ctrl Pts',(-145.859521458148,0.,35.0000000000001));
#9621=CARTESIAN_POINT('Ctrl Pts',(-138.765903145092,1.29386700370264,35.0000000000001));
#9622=CARTESIAN_POINT('Ctrl Pts',(-132.060245856224,2.98146159866235,35.0000000000001));
#9623=CARTESIAN_POINT('Ctrl Pts',(-125.680065601258,5.00000000000191,35.0000000000001));
#9624=CARTESIAN_POINT('',(-37.,59.9327136539873,35.0000000000001));
#9625=CARTESIAN_POINT('',(-36.8276756314269,0.,133.982075177761));
#9626=CARTESIAN_POINT('Ctrl Pts',(-125.680065601258,5.00000000000191,35.0000000000001));
#9627=CARTESIAN_POINT('Ctrl Pts',(-89.4344921386844,16.4672437124101,35.0000000000001));
#9628=CARTESIAN_POINT('Ctrl Pts',(-63.6931530394722,38.6151528519028,35.0000000000001));
#9629=CARTESIAN_POINT('Ctrl Pts',(-37.,59.9327136539873,35.0000000000001));
#9630=CARTESIAN_POINT('Ctrl Pts',(37.,59.9327136539873,35.0000000000001));
#9631=CARTESIAN_POINT('Ctrl Pts',(36.8276756314269,0.,133.982075177761));
#9632=CARTESIAN_POINT('Ctrl Pts',(35.9620587845551,61.072632135455,35.0000000000001));
#9633=CARTESIAN_POINT('Ctrl Pts',(36.6797497079439,0.,135.50941492147));
#9634=CARTESIAN_POINT('Ctrl Pts',(34.8494287906845,62.1881303927957,35.0000000000001));
#9635=CARTESIAN_POINT('Ctrl Pts',(36.4288634825457,0.,137.114741394618));
#9636=CARTESIAN_POINT('Ctrl Pts',(32.4772932645476,64.3449801372208,35.0000000000001));
#9637=CARTESIAN_POINT('Ctrl Pts',(35.6522781598644,0.,140.458171883983));
#9638=CARTESIAN_POINT('Ctrl Pts',(31.2177877322813,65.3863316243053,35.0000000000001));
#9639=CARTESIAN_POINT('Ctrl Pts',(35.126304365244,0.,142.196602013066));
#9640=CARTESIAN_POINT('Ctrl Pts',(28.5544031478084,67.3695815062162,35.0000000000001));
#9641=CARTESIAN_POINT('Ctrl Pts',(33.7243968013906,0.,145.755475174581));
#9642=CARTESIAN_POINT('Ctrl Pts',(27.1503938737515,68.3111074622806,35.0000000000001));
#9643=CARTESIAN_POINT('Ctrl Pts',(32.8479279009937,0.,147.576162799206));
#9644=CARTESIAN_POINT('Ctrl Pts',(24.2115292157522,70.0684707648054,35.0000000000001));
#9645=CARTESIAN_POINT('Ctrl Pts',(30.6756944321254,0.,151.21152369499));
#9646=CARTESIAN_POINT('Ctrl Pts',(22.6766738318099,70.8843081112658,35.0000000000001));
#9647=CARTESIAN_POINT('Ctrl Pts',(29.3791356772816,0.,153.026147945389));
#9648=CARTESIAN_POINT('Ctrl Pts',(19.4899048077957,72.3648035547606,35.0000000000001));
#9649=CARTESIAN_POINT('Ctrl Pts',(26.3232861859243,0.,156.52024682087));
#9650=CARTESIAN_POINT('Ctrl Pts',(17.8381180298111,73.0290133496626,35.0000000000001));
#9651=CARTESIAN_POINT('Ctrl Pts',(24.5631346628349,0.,158.199131371192));
#9652=CARTESIAN_POINT('Ctrl Pts',(14.4429405853757,74.1860012886773,35.0000000000001));
#9653=CARTESIAN_POINT('Ctrl Pts',(20.588388315684,0.,161.260182463203));
#9654=CARTESIAN_POINT('Ctrl Pts',(12.6995499189249,74.6787794327899,35.0000000000001));
#9655=CARTESIAN_POINT('Ctrl Pts',(18.3733019437227,0.,162.641132549651));
#9656=CARTESIAN_POINT('Ctrl Pts',(9.14636534104553,75.4735482731269,35.0000000000001));
#9657=CARTESIAN_POINT('Ctrl Pts',(13.5708791634494,0.,164.939399906875));
#9658=CARTESIAN_POINT('Ctrl Pts',(7.33698151150071,75.775223998754,35.0000000000001));
#9659=CARTESIAN_POINT('Ctrl Pts',(10.9839174320016,0.,165.855200551742));
#9660=CARTESIAN_POINT('Ctrl Pts',(3.68515441892942,76.1798832399239,35.0000000000001));
#9661=CARTESIAN_POINT('Ctrl Pts',(5.59736284229459,0.,167.093663864962));
#9662=CARTESIAN_POINT('Ctrl Pts',(1.84271115590295,76.2828667554667,35.0000000000001));
#9663=CARTESIAN_POINT('Ctrl Pts',(2.79913386299198,0.,167.415240784856));
#9664=CARTESIAN_POINT('Ctrl Pts',(-1.84271115590294,76.2828667554667,35.0000000000001));
#9665=CARTESIAN_POINT('Ctrl Pts',(-2.79913386299196,0.,167.415240784856));
#9666=CARTESIAN_POINT('Ctrl Pts',(-3.68515441892941,76.1798832399239,35.0000000000001));
#9667=CARTESIAN_POINT('Ctrl Pts',(-5.59736284229456,0.,167.093663864962));
#9668=CARTESIAN_POINT('Ctrl Pts',(-7.3369815115007,75.775223998754,35.0000000000001));
#9669=CARTESIAN_POINT('Ctrl Pts',(-10.9839174320016,0.,165.855200551742));
#9670=CARTESIAN_POINT('Ctrl Pts',(-9.14636534104552,75.4735482731269,35.0000000000001));
#9671=CARTESIAN_POINT('Ctrl Pts',(-13.5708791634494,0.,164.939399906875));
#9672=CARTESIAN_POINT('Ctrl Pts',(-12.6995499189248,74.6787794327899,35.0000000000001));
#9673=CARTESIAN_POINT('Ctrl Pts',(-18.3733019437227,0.,162.641132549651));
#9674=CARTESIAN_POINT('Ctrl Pts',(-14.4429405853757,74.1860012886772,35.0000000000001));
#9675=CARTESIAN_POINT('Ctrl Pts',(-20.5883883156839,0.,161.260182463203));
#9676=CARTESIAN_POINT('Ctrl Pts',(-17.8381180298111,73.0290133496626,35.0000000000001));
#9677=CARTESIAN_POINT('Ctrl Pts',(-24.5631346628349,0.,158.199131371192));
#9678=CARTESIAN_POINT('Ctrl Pts',(-19.4899048077957,72.3648035547606,35.0000000000001));
#9679=CARTESIAN_POINT('Ctrl Pts',(-26.3232861859242,0.,156.52024682087));
#9680=CARTESIAN_POINT('Ctrl Pts',(-22.6766738318099,70.8843081112658,35.0000000000001));
#9681=CARTESIAN_POINT('Ctrl Pts',(-29.3791356772816,0.,153.026147945389));
#9682=CARTESIAN_POINT('Ctrl Pts',(-24.2115292157522,70.0684707648055,35.0000000000001));
#9683=CARTESIAN_POINT('Ctrl Pts',(-30.6756944321254,0.,151.21152369499));
#9684=CARTESIAN_POINT('Ctrl Pts',(-27.1503938737515,68.3111074622806,35.0000000000001));
#9685=CARTESIAN_POINT('Ctrl Pts',(-32.8479279009936,0.,147.576162799206));
#9686=CARTESIAN_POINT('Ctrl Pts',(-28.5544031478084,67.3695815062162,35.0000000000001));
#9687=CARTESIAN_POINT('Ctrl Pts',(-33.7243968013906,0.,145.755475174581));
#9688=CARTESIAN_POINT('Ctrl Pts',(-31.2177877322813,65.3863316243053,35.0000000000001));
#9689=CARTESIAN_POINT('Ctrl Pts',(-35.126304365244,0.,142.196602013066));
#9690=CARTESIAN_POINT('Ctrl Pts',(-32.4772932645476,64.3449801372208,35.0000000000001));
#9691=CARTESIAN_POINT('Ctrl Pts',(-35.6522781598644,0.,140.458171883983));
#9692=CARTESIAN_POINT('Ctrl Pts',(-34.8494287906845,62.1881303927957,35.0000000000001));
#9693=CARTESIAN_POINT('Ctrl Pts',(-36.4288634825457,0.,137.114741394618));
#9694=CARTESIAN_POINT('Ctrl Pts',(-35.9620587845551,61.0726321354551,35.0000000000001));
#9695=CARTESIAN_POINT('Ctrl Pts',(-36.6797497079439,0.,135.50941492147));
#9696=CARTESIAN_POINT('Ctrl Pts',(-37.,59.9327136539873,35.0000000000001));
#9697=CARTESIAN_POINT('Ctrl Pts',(-36.8276756314269,0.,133.982075177761));
#9698=CARTESIAN_POINT('Ctrl Pts',(-37.,59.9327136539873,35.0000000000001));
#9699=CARTESIAN_POINT('Ctrl Pts',(-34.9241175691101,62.2125506169229,35.0000000000001));
#9700=CARTESIAN_POINT('Ctrl Pts',(-32.5494800245177,64.3947066833499,35.0000000000001));
#9701=CARTESIAN_POINT('Ctrl Pts',(-29.8860954400449,66.3779565652608,35.0000000000001));
#9702=CARTESIAN_POINT('Ctrl Pts',(-27.222710855572,68.3612064471716,35.0000000000001));
#9703=CARTESIAN_POINT('Ctrl Pts',(-24.270058343817,70.1440603895185,35.0000000000001));
#9704=CARTESIAN_POINT('Ctrl Pts',(-21.0832893198028,71.6245558330132,35.0000000000001));
#9705=CARTESIAN_POINT('Ctrl Pts',(-17.8965202957886,73.105051276508,35.0000000000001));
#9706=CARTESIAN_POINT('Ctrl Pts',(-14.4761422078645,74.2813950126213,35.0000000000001));
#9707=CARTESIAN_POINT('Ctrl Pts',(-10.9229576299852,75.0761638529584,35.0000000000001));
#9708=CARTESIAN_POINT('Ctrl Pts',(-7.36977305210586,75.8709326932955,35.0000000000001));
#9709=CARTESIAN_POINT('Ctrl Pts',(-3.68542231180589,76.2828667554667,35.0000000000001));
#9710=CARTESIAN_POINT('Ctrl Pts',(8.60422844084496E-15,76.2828667554667,
35.0000000000001));
#9711=CARTESIAN_POINT('Ctrl Pts',(3.68542231180591,76.2828667554667,35.0000000000001));
#9712=CARTESIAN_POINT('Ctrl Pts',(7.36977305210588,75.8709326932955,35.0000000000001));
#9713=CARTESIAN_POINT('Ctrl Pts',(10.9229576299852,75.0761638529584,35.0000000000001));
#9714=CARTESIAN_POINT('Ctrl Pts',(14.4761422078645,74.2813950126214,35.0000000000001));
#9715=CARTESIAN_POINT('Ctrl Pts',(17.8965202957886,73.105051276508,35.0000000000001));
#9716=CARTESIAN_POINT('Ctrl Pts',(21.0832893198028,71.6245558330132,35.0000000000001));
#9717=CARTESIAN_POINT('Ctrl Pts',(24.2700583438171,70.1440603895185,35.0000000000001));
#9718=CARTESIAN_POINT('Ctrl Pts',(27.222710855572,68.3612064471716,35.0000000000001));
#9719=CARTESIAN_POINT('Ctrl Pts',(29.8860954400449,66.3779565652607,35.0000000000001));
#9720=CARTESIAN_POINT('Ctrl Pts',(32.5494800245177,64.3947066833499,35.0000000000001));
#9721=CARTESIAN_POINT('Ctrl Pts',(34.9241175691101,62.2125506169228,35.0000000000001));
#9722=CARTESIAN_POINT('Ctrl Pts',(37.,59.9327136539873,35.0000000000001));
#9723=CARTESIAN_POINT('Ctrl Pts',(-126.333741430004,4.79470864688834,25.0000000000001));
#9724=CARTESIAN_POINT('Ctrl Pts',(-126.333741430004,4.79470864688834,37.0000000000001));
#9725=CARTESIAN_POINT('Ctrl Pts',(-89.7434098754838,16.201390763878,25.0000000000001));
#9726=CARTESIAN_POINT('Ctrl Pts',(-89.7434098754838,16.201390763878,37.0000000000001));
#9727=CARTESIAN_POINT('Ctrl Pts',(-63.8533409646905,38.4872243216708,25.0000000000001));
#9728=CARTESIAN_POINT('Ctrl Pts',(-63.8533409646905,38.4872243216708,37.0000000000001));
#9729=CARTESIAN_POINT('Ctrl Pts',(-37.,59.9327136539873,25.0000000000001));
#9730=CARTESIAN_POINT('Ctrl Pts',(-37.,59.9327136539873,37.0000000000001));
#9731=CARTESIAN_POINT('',(-37.,59.9327136539873,25.0000000000001));
#9732=CARTESIAN_POINT('Origin',(5.94655548926424E-16,26.2427388041954,25.0000000000001));
#9733=CARTESIAN_POINT('',(20.,72.1122755947453,-11.9999999999999));
#9734=CARTESIAN_POINT('Ctrl Pts',(-20.,72.1122755947453,-11.9999999999999));
#9735=CARTESIAN_POINT('Ctrl Pts',(-20.,72.1122755947453,-10.7281705881235));
#9736=CARTESIAN_POINT('Ctrl Pts',(-19.876740954423,72.1666695578122,-9.41819722511157));
#9737=CARTESIAN_POINT('Ctrl Pts',(-19.363419845374,72.3854545732174,-6.82230663106049));
#9738=CARTESIAN_POINT('Ctrl Pts',(-18.9735260730669,72.5495796554118,-5.53633371502868));
#9739=CARTESIAN_POINT('Ctrl Pts',(-17.9489707104667,72.9562551485406,-3.07765863937579));
#9740=CARTESIAN_POINT('Ctrl Pts',(-17.3134969066183,73.1986589652098,-1.90272848601112));
#9741=CARTESIAN_POINT('Ctrl Pts',(-15.8503625531969,73.7125357294074,0.266950487449766));
#9742=CARTESIAN_POINT('Ctrl Pts',(-15.0225516277294,73.9834946181185,1.26171961973252));
#9743=CARTESIAN_POINT('Ctrl Pts',(-13.2626071807075,74.5020216025358,3.02166406675442));
#9744=CARTESIAN_POINT('Ctrl Pts',(-12.2682645673177,74.7684339328333,3.84936166480408));
#9745=CARTESIAN_POINT('Ctrl Pts',(-10.0983665793023,75.2659618277825,5.31287304805954));
#9746=CARTESIAN_POINT('Ctrl Pts',(-8.92278917997,75.4966497262723,5.94879953171039));
#9747=CARTESIAN_POINT('Ctrl Pts',(-6.46280366693619,75.8793792723685,6.97387010022773));
#9748=CARTESIAN_POINT('Ctrl Pts',(-5.17618585589729,76.0314587231336,7.36382898538741));
#9749=CARTESIAN_POINT('Ctrl Pts',(-2.58007773937013,76.2332652071209,7.87697089230036));
#9750=CARTESIAN_POINT('Ctrl Pts',(-1.2705472609979,76.2828667554667,8.00000000000007));
#9751=CARTESIAN_POINT('Ctrl Pts',(1.2705472609979,76.2828667554667,8.00000000000007));
#9752=CARTESIAN_POINT('Ctrl Pts',(2.58007773937013,76.2332652071209,7.87697089230036));
#9753=CARTESIAN_POINT('Ctrl Pts',(5.17618585589729,76.0314587231336,7.36382898538741));
#9754=CARTESIAN_POINT('Ctrl Pts',(6.46280366693619,75.8793792723685,6.97387010022773));
#9755=CARTESIAN_POINT('Ctrl Pts',(8.92278917997,75.4966497262723,5.94879953171039));
#9756=CARTESIAN_POINT('Ctrl Pts',(10.0983665793023,75.2659618277825,5.31287304805954));
#9757=CARTESIAN_POINT('Ctrl Pts',(12.2682645673177,74.7684339328333,3.84936166480408));
#9758=CARTESIAN_POINT('Ctrl Pts',(13.2626071807075,74.5020216025358,3.02166406675442));
#9759=CARTESIAN_POINT('Ctrl Pts',(15.0225516277294,73.9834946181185,1.26171961973252));
#9760=CARTESIAN_POINT('Ctrl Pts',(15.8503625531969,73.7125357294074,0.266950487449763));
#9761=CARTESIAN_POINT('Ctrl Pts',(17.3134969066183,73.1986589652098,-1.90272848601112));
#9762=CARTESIAN_POINT('Ctrl Pts',(17.9489707104667,72.9562551485406,-3.07765863937579));
#9763=CARTESIAN_POINT('Ctrl Pts',(18.9735260730669,72.5495796554118,-5.53633371502868));
#9764=CARTESIAN_POINT('Ctrl Pts',(19.363419845374,72.3854545732174,-6.82230663106049));
#9765=CARTESIAN_POINT('Ctrl Pts',(19.876740954423,72.1666695578122,-9.41819722511157));
#9766=CARTESIAN_POINT('Ctrl Pts',(20.,72.1122755947453,-10.7281705881235));
#9767=CARTESIAN_POINT('Ctrl Pts',(20.,72.1122755947453,-11.9999999999999));
#9768=CARTESIAN_POINT('',(-20.,72.1122755947453,-11.9999999999999));
#9769=CARTESIAN_POINT('',(37.,59.9327136539873,25.0000000000001));
#9770=CARTESIAN_POINT('Ctrl Pts',(37.,59.9327136539873,25.0000000000001));
#9771=CARTESIAN_POINT('Ctrl Pts',(37.,59.9327136539873,37.0000000000001));
#9772=CARTESIAN_POINT('Ctrl Pts',(63.8533446476634,38.4872213803922,25.0000000000001));
#9773=CARTESIAN_POINT('Ctrl Pts',(63.8533446476634,38.4872213803922,37.0000000000001));
#9774=CARTESIAN_POINT('Ctrl Pts',(89.7434169772014,16.2013846508122,25.0000000000001));
#9775=CARTESIAN_POINT('Ctrl Pts',(89.7434169772014,16.2013846508122,37.0000000000001));
#9776=CARTESIAN_POINT('Ctrl Pts',(126.333756485248,4.79470395356222,25.0000000000001));
#9777=CARTESIAN_POINT('Ctrl Pts',(126.333756485248,4.79470395356222,37.0000000000001));
#9778=CARTESIAN_POINT('Origin',(37.,-5.,35.0000000000001));
#9779=CARTESIAN_POINT('',(-145.859521458148,0.,35.0000000000001));
#9780=CARTESIAN_POINT('Origin',(37.,-5.,35.0000000000001));
#9781=CARTESIAN_POINT('',(145.859521458148,0.,35.0000000000001));
#9782=CARTESIAN_POINT('Origin',(-99.7519848385422,-5.,-11.9999999999999));
#9783=CARTESIAN_POINT('',(-145.859521458148,-5.,-58.9999999999999));
#9784=CARTESIAN_POINT('Origin',(99.7519848385422,-5.,-11.9999999999999));
#9785=CARTESIAN_POINT('',(145.859521458148,-5.,-59.));
#9786=CARTESIAN_POINT('Origin',(-145.859521458148,-4.99999999999993,-168.542028553823));
#9787=CARTESIAN_POINT('',(-36.827675631427,6.20110919257889E-14,-157.982075177761));
#9788=CARTESIAN_POINT('Ctrl Pts',(-145.859521458148,1.99232991215936E-14,
-58.9999999999999));
#9789=CARTESIAN_POINT('Ctrl Pts',(-145.635702363347,0.000231282966572025,
-58.9999999999999));
#9790=CARTESIAN_POINT('Ctrl Pts',(-145.411883254566,0.000447783515656521,
-59.0006859694108));
#9791=CARTESIAN_POINT('Ctrl Pts',(-145.18806728541,0.000650024995078429,
-59.0020579084895));
#9792=CARTESIAN_POINT('Ctrl Pts',(-139.052999251965,0.00619371001492337,
-59.039664427889));
#9793=CARTESIAN_POINT('Ctrl Pts',(-132.962545443942,9.41456194013237E-14,
-59.592285658951));
#9794=CARTESIAN_POINT('Ctrl Pts',(-126.977116946521,7.40439610666388E-14,
-60.6397078209218));
#9795=CARTESIAN_POINT('Ctrl Pts',(-123.729336577931,6.46076837229338E-14,
-61.208054287134));
#9796=CARTESIAN_POINT('Ctrl Pts',(-120.512481495564,9.59966811121834E-14,
-61.9221153240676));
#9797=CARTESIAN_POINT('Ctrl Pts',(-117.336234309904,9.53981529460291E-14,
-62.7787168150854));
#9798=CARTESIAN_POINT('Ctrl Pts',(-114.085205078271,1.09954677696283E-13,
-63.6554862616612));
#9799=CARTESIAN_POINT('Ctrl Pts',(-110.876720955829,3.88437234764698E-14,
-64.6815897913564));
#9800=CARTESIAN_POINT('Ctrl Pts',(-107.721164151354,6.31408343849688E-14,
-65.8535592808521));
#9801=CARTESIAN_POINT('Ctrl Pts',(-104.510754540394,7.27076390459741E-14,
-67.0459010277961));
#9802=CARTESIAN_POINT('Ctrl Pts',(-101.355129960864,2.13060038867633E-14,
-68.3892216824963));
#9803=CARTESIAN_POINT('Ctrl Pts',(-98.2651875381796,7.99960446463358E-14,
-69.8797997202865));
#9804=CARTESIAN_POINT('Ctrl Pts',(-95.141608011939,1.21775280556001E-13,
-71.3866041859377));
#9805=CARTESIAN_POINT('Ctrl Pts',(-92.0851458120254,4.16371041647899E-14,
-73.0438828741871));
#9806=CARTESIAN_POINT('Ctrl Pts',(-89.1070253835134,5.55641162014496E-14,
-74.847790689453));
#9807=CARTESIAN_POINT('Ctrl Pts',(-86.1168527340016,6.74633771530896E-14,
-76.6589987788935));
#9808=CARTESIAN_POINT('Ctrl Pts',(-83.2056472832252,1.97565378180188E-14,
-78.6180166790309));
#9809=CARTESIAN_POINT('Ctrl Pts',(-80.384830163582,3.31094929983044E-14,
-80.7210696683278));
#9810=CARTESIAN_POINT('Ctrl Pts',(-77.5611534148132,3.07519208876647E-14,
-82.8262546468059));
#9811=CARTESIAN_POINT('Ctrl Pts',(-74.8381140101429,6.55809408055033E-14,
-85.0685191399763));
#9812=CARTESIAN_POINT('Ctrl Pts',(-72.2297132774974,2.94546559451853E-14,
-87.4364962704631));
#9813=CARTESIAN_POINT('Ctrl Pts',(-69.6213194790229,1.09983012374116E-14,
-89.8044671059209));
#9814=CARTESIAN_POINT('Ctrl Pts',(-67.1275347240066,2.00661256494869E-14,
-92.2980716005061));
#9815=CARTESIAN_POINT('Ctrl Pts',(-64.7594023581046,4.44089209850063E-15,
-94.9062580231543));
#9816=CARTESIAN_POINT('Ctrl Pts',(-62.402101299093,1.71643312990407E-14,
-97.5025151854376));
#9817=CARTESIAN_POINT('Ctrl Pts',(-60.1698465605611,7.92727737594203E-14,
-100.211731774115));
#9818=CARTESIAN_POINT('Ctrl Pts',(-58.0726499521868,5.06167238114794E-14,
-103.021640804036));
#9819=CARTESIAN_POINT('Ctrl Pts',(-55.994832850032,1.08718014075603E-14,
-105.805584385938));
#9820=CARTESIAN_POINT('Ctrl Pts',(-54.0490749518659,-5.23372399894248E-14,
-108.689139472133));
#9821=CARTESIAN_POINT('Ctrl Pts',(-52.2449416359333,8.70188233993832E-15,
-111.658230646188));
#9822=CARTESIAN_POINT('Ctrl Pts',(-50.4652489916242,4.61267413567307E-14,
-114.587099414412));
#9823=CARTESIAN_POINT('Ctrl Pts',(-48.8232383526353,-3.96485956199284E-15,
-117.599305307977));
#9824=CARTESIAN_POINT('Ctrl Pts',(-47.3258881353928,-1.91641373722875E-14,
-120.682033527671));
#9825=CARTESIAN_POINT('Ctrl Pts',(-45.8550866032242,-8.76261135605058E-15,
-123.710103605448));
#9826=CARTESIAN_POINT('Ctrl Pts',(-44.5237168473911,9.44160675302571E-16,
-126.806759783349));
#9827=CARTESIAN_POINT('Ctrl Pts',(-43.3384647873199,3.63520113533591E-14,
-129.955904638828));
#9828=CARTESIAN_POINT('Ctrl Pts',(-42.178411369753,8.22686500091128E-14,
-133.03809818658));
#9829=CARTESIAN_POINT('Ctrl Pts',(-41.1578799651058,2.73842972706966E-14,
-136.171204882295));
#9830=CARTESIAN_POINT('Ctrl Pts',(-40.2800279987793,2.40516445328869E-14,
-139.345683225176));
#9831=CARTESIAN_POINT('Ctrl Pts',(-38.5944013814791,-4.43847532318893E-14,
-145.441227116471));
#9832=CARTESIAN_POINT('Ctrl Pts',(-37.4373840532588,1.49418878328148E-13,
-151.68681682945));
#9833=CARTESIAN_POINT('Ctrl Pts',(-36.827675631427,5.35189297393157E-14,
-157.982075177761));
#9834=CARTESIAN_POINT('',(-36.827675631427,-4.99999999999994,-157.982075177761));
#9835=CARTESIAN_POINT('Origin',(145.859521458148,-4.99999999999993,-168.542028553823));
#9836=CARTESIAN_POINT('',(36.8276756314269,6.20110919257889E-14,-157.98207517776));
#9837=CARTESIAN_POINT('Ctrl Pts',(145.859521458148,1.99966320462804E-14,
-59.));
#9838=CARTESIAN_POINT('Ctrl Pts',(145.635702363798,0.000231282957399252,
-59.));
#9839=CARTESIAN_POINT('Ctrl Pts',(145.411883255443,0.000447783508952677,
-59.0006859694082));
#9840=CARTESIAN_POINT('Ctrl Pts',(145.188067286725,0.000650024989461163,
-59.0020579084816));
#9841=CARTESIAN_POINT('Ctrl Pts',(139.052999252887,0.00619371005042004,
-59.0396644278098));
#9842=CARTESIAN_POINT('Ctrl Pts',(132.962545444417,-1.11887795632077E-13,
-59.592285658868));
#9843=CARTESIAN_POINT('Ctrl Pts',(126.977116946521,-1.04423077240787E-13,
-60.639707820922));
#9844=CARTESIAN_POINT('Ctrl Pts',(123.729336577944,-9.67014244773527E-14,
-61.2080542871319));
#9845=CARTESIAN_POINT('Ctrl Pts',(120.512481495576,-1.13587683266672E-13,
-61.9221153240646));
#9846=CARTESIAN_POINT('Ctrl Pts',(117.336234309904,-6.90972208920379E-14,
-62.7787168150856));
#9847=CARTESIAN_POINT('Ctrl Pts',(114.085205078283,-2.10873246295173E-14,
-63.6554862616581));
#9848=CARTESIAN_POINT('Ctrl Pts',(110.87672095584,-5.77851871173568E-14,
-64.6815897913523));
#9849=CARTESIAN_POINT('Ctrl Pts',(107.721164151354,-7.0435270368486E-14,
-65.8535592808523));
#9850=CARTESIAN_POINT('Ctrl Pts',(104.510754540406,-5.9941934650156E-14,
-67.0459010277919));
#9851=CARTESIAN_POINT('Ctrl Pts',(101.355129960875,-7.52622445179423E-14,
-68.389221682491));
#9852=CARTESIAN_POINT('Ctrl Pts',(98.2651875381795,-6.59048807687785E-14,
-69.8797997202867));
#9853=CARTESIAN_POINT('Ctrl Pts',(95.1416080119508,-2.09429382763629E-14,
-71.3866041859322));
#9854=CARTESIAN_POINT('Ctrl Pts',(92.0851458120368,-4.4049120057977E-14,
-73.0438828741804));
#9855=CARTESIAN_POINT('Ctrl Pts',(89.1070253835134,-1.83922193067957E-14,
-74.8477906894531));
#9856=CARTESIAN_POINT('Ctrl Pts',(86.1168527340136,-2.8634501446293E-14,
-76.6589987788863));
#9857=CARTESIAN_POINT('Ctrl Pts',(83.2056472832369,1.40408434793159E-14,
-78.6180166790223));
#9858=CARTESIAN_POINT('Ctrl Pts',(80.3848301635821,-1.04201332750223E-14,
-80.7210696683279));
#9859=CARTESIAN_POINT('Ctrl Pts',(77.561153414816,-2.03746625468862E-14,
-82.8262546468039));
#9860=CARTESIAN_POINT('Ctrl Pts',(74.8381140101453,-3.84257827749966E-14,
-85.0685191399742));
#9861=CARTESIAN_POINT('Ctrl Pts',(72.2297132774974,-4.91540503775017E-14,
-87.4364962704632));
#9862=CARTESIAN_POINT('Ctrl Pts',(69.6213194790202,-3.34285257340705E-14,
-89.8044671059234));
#9863=CARTESIAN_POINT('Ctrl Pts',(67.1275347240061,-1.45705862260143E-14,
-92.2980716005068));
#9864=CARTESIAN_POINT('Ctrl Pts',(64.7594023581046,-1.87525810038756E-14,
-94.9062580231544));
#9865=CARTESIAN_POINT('Ctrl Pts',(62.4021012990951,-1.76400073832052E-14,
-97.5025151854354));
#9866=CARTESIAN_POINT('Ctrl Pts',(60.1698465605618,-7.19881477211928E-14,
-100.211731774114));
#9867=CARTESIAN_POINT('Ctrl Pts',(58.0726499521868,-5.42214207492858E-14,
-103.021640804037));
#9868=CARTESIAN_POINT('Ctrl Pts',(55.994832850029,-2.90803087727514E-14,
-105.805584385943));
#9869=CARTESIAN_POINT('Ctrl Pts',(54.0490749518629,-7.79522172356907E-14,
-108.689139472138));
#9870=CARTESIAN_POINT('Ctrl Pts',(52.2449416359332,-1.01288911340345E-13,
-111.658230646188));
#9871=CARTESIAN_POINT('Ctrl Pts',(50.4652489916246,-1.2018699629012E-13,
-114.587099414412));
#9872=CARTESIAN_POINT('Ctrl Pts',(48.8232383526351,-2.65689998570122E-14,
-117.599305307977));
#9873=CARTESIAN_POINT('Ctrl Pts',(47.3258881353929,-8.66874694043732E-16,
-120.682033527671));
#9874=CARTESIAN_POINT('Ctrl Pts',(45.855086603224,4.04340402343437E-14,
-123.710103605448));
#9875=CARTESIAN_POINT('Ctrl Pts',(44.5237168473911,-2.2235983896746E-14,
-126.806759783349));
#9876=CARTESIAN_POINT('Ctrl Pts',(43.3384647873198,-8.23114176779849E-14,
-129.955904638828));
#9877=CARTESIAN_POINT('Ctrl Pts',(42.1784113697529,-1.68925830949098E-13,
-133.03809818658));
#9878=CARTESIAN_POINT('Ctrl Pts',(41.1578799651058,-8.85986346721827E-14,
-136.171204882295));
#9879=CARTESIAN_POINT('Ctrl Pts',(40.2800279987792,-4.7668540935266E-14,
-139.345683225176));
#9880=CARTESIAN_POINT('Ctrl Pts',(38.5944013814802,5.17415891553732E-14,
-145.441227116467));
#9881=CARTESIAN_POINT('Ctrl Pts',(37.4373840532589,8.01494831266999E-14,
-151.686816829449));
#9882=CARTESIAN_POINT('Ctrl Pts',(36.8276756314269,-5.35238086490919E-14,
-157.982075177761));
#9883=CARTESIAN_POINT('',(36.8276756314269,-4.99999999999994,-157.982075177761));
#9884=CARTESIAN_POINT('Origin',(-5.2737622621639E-14,-4.99999999999994,
-154.415240784856));
#9885=CARTESIAN_POINT('Ctrl Pts',(-36.827675631427,6.00431163122472E-14,
-157.982075177761));
#9886=CARTESIAN_POINT('Ctrl Pts',(-36.679749707944,6.07211040707748E-14,
-159.50941492147));
#9887=CARTESIAN_POINT('Ctrl Pts',(-36.4288634825458,6.14323406959253E-14,
-161.114741394618));
#9888=CARTESIAN_POINT('Ctrl Pts',(-36.0405708212051,6.21724893790088E-14,
-162.786456639301));
#9889=CARTESIAN_POINT('Ctrl Pts',(-35.6522781598644,6.07095392476017E-14,
-164.458171883983));
#9890=CARTESIAN_POINT('Ctrl Pts',(-35.1263043652441,6.14323406959253E-14,
-166.196602013066));
#9891=CARTESIAN_POINT('Ctrl Pts',(-34.4253505833174,6.21724893790088E-14,
-167.976038593823));
#9892=CARTESIAN_POINT('Ctrl Pts',(-33.7243968013906,6.95739762098431E-14,
-169.755475174581));
#9893=CARTESIAN_POINT('Ctrl Pts',(-32.8479279009937,7.03141248929266E-14,
-171.576162799206));
#9894=CARTESIAN_POINT('Ctrl Pts',(-31.7618111665596,7.105427357601E-14,
-173.393843247098));
#9895=CARTESIAN_POINT('Ctrl Pts',(-30.6756944321255,6.95508465634968E-14,
-175.21152369499));
#9896=CARTESIAN_POINT('Ctrl Pts',(-29.3791356772817,7.03141248929266E-14,
-177.026147945389));
#9897=CARTESIAN_POINT('Ctrl Pts',(-27.851210931603,7.105427357601E-14,-178.773197383129));
#9898=CARTESIAN_POINT('Ctrl Pts',(-26.3232861859243,6.96896244415749E-14,
-180.520246820869));
#9899=CARTESIAN_POINT('Ctrl Pts',(-24.563134662835,7.0406643478312E-14,
-182.199131371192));
#9900=CARTESIAN_POINT('Ctrl Pts',(-22.5757614892595,7.105427357601E-14,
-183.729656917197));
#9901=CARTESIAN_POINT('Ctrl Pts',(-20.588388315684,7.00250043135971E-14,
-185.260182463203));
#9902=CARTESIAN_POINT('Ctrl Pts',(-18.3733019437227,7.05916806490829E-14,
-186.64113254965));
#9903=CARTESIAN_POINT('Ctrl Pts',(-15.9720905535861,7.105427357601E-14,
-187.790266228263));
#9904=CARTESIAN_POINT('Ctrl Pts',(-13.5708791634495,7.92652980289669E-14,
-188.939399906875));
#9905=CARTESIAN_POINT('Ctrl Pts',(-10.9839174320017,7.9658502016855E-14,
-189.855200551742));
#9906=CARTESIAN_POINT('Ctrl Pts',(-8.29064013714815,7.99360577730113E-14,
-190.474432208352));
#9907=CARTESIAN_POINT('Ctrl Pts',(-5.59736284229463,7.97972798949331E-14,
-191.093663864962));
#9908=CARTESIAN_POINT('Ctrl Pts',(-2.79913386299203,7.99360577730113E-14,
-191.415240784856));
#9909=CARTESIAN_POINT('Ctrl Pts',(-5.19029264012261E-14,7.99360577730113E-14,
-191.415240784856));
#9910=CARTESIAN_POINT('Ctrl Pts',(2.79913386299191,8.03755210535921E-14,
-191.415240784856));
#9911=CARTESIAN_POINT('Ctrl Pts',(5.59736284229452,8.02136135291676E-14,
-191.093663864962));
#9912=CARTESIAN_POINT('Ctrl Pts',(8.29064013714802,7.99360577730113E-14,
-190.474432208352));
#9913=CARTESIAN_POINT('Ctrl Pts',(10.9839174320015,7.18753760213057E-14,
-189.855200551742));
#9914=CARTESIAN_POINT('Ctrl Pts',(13.5708791634494,7.15168665029372E-14,
-188.939399906875));
#9915=CARTESIAN_POINT('Ctrl Pts',(15.972090553586,7.105427357601E-14,-187.790266228263));
#9916=CARTESIAN_POINT('Ctrl Pts',(18.3733019437226,7.2280144832367E-14,
-186.64113254965));
#9917=CARTESIAN_POINT('Ctrl Pts',(20.5883883156839,7.1701903673708E-14,
-185.260182463203));
#9918=CARTESIAN_POINT('Ctrl Pts',(22.5757614892594,7.105427357601E-14,-183.729656917197));
#9919=CARTESIAN_POINT('Ctrl Pts',(24.5631346628349,7.25114412958305E-14,
-182.199131371191));
#9920=CARTESIAN_POINT('Ctrl Pts',(26.3232861859242,7.17944222590935E-14,
-180.520246820869));
#9921=CARTESIAN_POINT('Ctrl Pts',(27.8512109316029,7.105427357601E-14,-178.773197383129));
#9922=CARTESIAN_POINT('Ctrl Pts',(29.3791356772816,7.25345709421769E-14,
-177.026147945389));
#9923=CARTESIAN_POINT('Ctrl Pts',(30.6756944321254,7.17944222590935E-14,
-175.21152369499));
#9924=CARTESIAN_POINT('Ctrl Pts',(31.7618111665595,7.105427357601E-14,-173.393843247098));
#9925=CARTESIAN_POINT('Ctrl Pts',(32.8479279009936,6.36701339799354E-14,
-171.576162799206));
#9926=CARTESIAN_POINT('Ctrl Pts',(33.7243968013905,6.29126380620922E-14,
-169.755475174581));
#9927=CARTESIAN_POINT('Ctrl Pts',(34.4253505833173,6.21724893790088E-14,
-167.976038593823));
#9928=CARTESIAN_POINT('Ctrl Pts',(35.126304365244,6.36816988031086E-14,
-166.196602013066));
#9929=CARTESIAN_POINT('Ctrl Pts',(35.6522781598643,6.29126380620922E-14,
-164.458171883983));
#9930=CARTESIAN_POINT('Ctrl Pts',(36.040570821205,6.21724893790088E-14,
-162.786456639301));
#9931=CARTESIAN_POINT('Ctrl Pts',(36.4288634825457,6.36874812146952E-14,
-161.114741394618));
#9932=CARTESIAN_POINT('Ctrl Pts',(36.6797497079439,6.29126380620922E-14,
-159.509414921469));
#9933=CARTESIAN_POINT('Ctrl Pts',(36.8276756314269,6.21724893790088E-14,
-157.98207517776));
#9934=CARTESIAN_POINT('Ctrl Pts',(145.859521458148,1.99966320462804E-14,
-59.));
#9935=CARTESIAN_POINT('Ctrl Pts',(145.859521458148,1.99966320462804E-14,
-59.));
#9936=CARTESIAN_POINT('Ctrl Pts',(139.935495507955,1.08053483677362,-59.));
#9937=CARTESIAN_POINT('Ctrl Pts',(139.721849114916,-0.00946396581249335,
-59.));
#9938=CARTESIAN_POINT('Ctrl Pts',(134.282043748658,2.43566561952013,-59.));
#9939=CARTESIAN_POINT('Ctrl Pts',(133.377109516276,-0.0213330059978996,
-59.5229040505835));
#9940=CARTESIAN_POINT('Ctrl Pts',(126.153138109028,4.82540450931204,-59.));
#9941=CARTESIAN_POINT('Ctrl Pts',(123.752347114045,-0.0422637584217218,
-61.2196520084283));
#9942=CARTESIAN_POINT('Ctrl Pts',(123.502048229037,5.68149125852136,-59.));
#9943=CARTESIAN_POINT('Ctrl Pts',(120.52689037285,-0.0497618745872814,-61.9367613521045));
#9944=CARTESIAN_POINT('Ctrl Pts',(118.307860920989,7.50353712828284,-59.));
#9945=CARTESIAN_POINT('Ctrl Pts',(114.083064303984,-0.0657204343980337,
-63.6868647700364));
#9946=CARTESIAN_POINT('Ctrl Pts',(115.764763492932,8.469496248835,-59.));
#9947=CARTESIAN_POINT('Ctrl Pts',(110.864745391586,-0.0741808780432265,
-64.7198997778734));
#9948=CARTESIAN_POINT('Ctrl Pts',(110.777462874248,10.5021449940676,-59.));
#9949=CARTESIAN_POINT('Ctrl Pts',(104.480363411824,-0.0919840229109741,
-67.1072738686291));
#9950=CARTESIAN_POINT('Ctrl Pts',(108.33325968362,11.5688346187481,-59.));
#9951=CARTESIAN_POINT('Ctrl Pts',(101.314363689722,-0.101326724133529,-68.4616401636748));
#9952=CARTESIAN_POINT('Ctrl Pts',(103.53464932529,13.7938025050227,-59.));
#9953=CARTESIAN_POINT('Ctrl Pts',(95.0816761557438,-0.12081431425373,-71.488542771471));
#9954=CARTESIAN_POINT('Ctrl Pts',(101.180242157587,14.9520807666169,-59.));
#9955=CARTESIAN_POINT('Ctrl Pts',(92.01506006982,-0.130959203151376,-73.1610880645267));
#9956=CARTESIAN_POINT('Ctrl Pts',(96.5521256306011,17.3510840595046,-59.));
#9957=CARTESIAN_POINT('Ctrl Pts',(86.0280376851247,-0.151971098719488,-76.8121020395858));
#9958=CARTESIAN_POINT('Ctrl Pts',(94.2784162713182,18.591809090798,-59.));
#9959=CARTESIAN_POINT('Ctrl Pts',(83.1077052322228,-0.162838105389954,-78.7905587679407));
#9960=CARTESIAN_POINT('Ctrl Pts',(89.8025971466679,21.1465640558695,-59.));
#9961=CARTESIAN_POINT('Ctrl Pts',(77.4577804203387,-0.185214166601435,-83.032072624605));
#9962=CARTESIAN_POINT('Ctrl Pts',(87.6004873813004,22.4605939896476,-59.));
#9963=CARTESIAN_POINT('Ctrl Pts',(74.7282568958346,-0.19672322114245,-85.2950966600411));
#9964=CARTESIAN_POINT('Ctrl Pts',(83.2587692299763,25.152816892474,-59.));
#9965=CARTESIAN_POINT('Ctrl Pts',(69.499944269098,-0.220303308192758,-90.0760233255031));
#9966=CARTESIAN_POINT('Ctrl Pts',(81.1191608440196,26.5310098615222,-59.));
#9967=CARTESIAN_POINT('Ctrl Pts',(67.0012121106908,-0.232374340702051,-92.5938742603756));
#9968=CARTESIAN_POINT('Ctrl Pts',(76.8933472370124,29.3424169676743,-59.));
#9969=CARTESIAN_POINT('Ctrl Pts',(62.2680278295026,-0.256998313786643,-97.8476184497509));
#9970=CARTESIAN_POINT('Ctrl Pts',(74.8071420159619,30.7756311047781,-59.));
#9971=CARTESIAN_POINT('Ctrl Pts',(60.0336152811755,-0.269551254361943,-100.58344638055));
#9972=CARTESIAN_POINT('Ctrl Pts',(70.6790365242624,33.6879386798268,-59.));
#9973=CARTESIAN_POINT('Ctrl Pts',(55.8546997830352,-0.295058973676278,-106.230970575318));
#9974=CARTESIAN_POINT('Ctrl Pts',(68.6371362536135,35.1670321177717,-59.));
#9975=CARTESIAN_POINT('Ctrl Pts',(53.9102158500078,-0.308013752415314,-109.142594489691));
#9976=CARTESIAN_POINT('Ctrl Pts',(64.5885424482124,38.1619564272879,-59.));
#9977=CARTESIAN_POINT('Ctrl Pts',(50.3279822597621,-0.33424507815485,-115.096290916415));
#9978=CARTESIAN_POINT('Ctrl Pts',(62.5818489134604,39.6777872988593,-59.));
#9979=CARTESIAN_POINT('Ctrl Pts',(48.690230578512,-0.34752162515535,-118.13829117116));
#9980=CARTESIAN_POINT('Ctrl Pts',(58.5945703653485,42.7370446084141,-59.));
#9981=CARTESIAN_POINT('Ctrl Pts',(45.7292271162558,-0.374316417515544,-124.306271647363));
#9982=CARTESIAN_POINT('Ctrl Pts',(56.6139853519887,44.2804710463975,-58.9999999999999));
#9983=CARTESIAN_POINT('Ctrl Pts',(44.4059543564031,-0.387834662875238,-127.432186195309));
#9984=CARTESIAN_POINT('Ctrl Pts',(52.6698256321568,47.3857776215616,-58.9999999999999));
#9985=CARTESIAN_POINT('Ctrl Pts',(42.0729707249933,-0.415032782051548,-133.722570987114));
#9986=CARTESIAN_POINT('Ctrl Pts',(50.7062509256847,48.9476577587424,-58.9999999999999));
#9987=CARTESIAN_POINT('Ctrl Pts',(41.0632239705788,-0.428712655868165,-136.88698710447));
#9988=CARTESIAN_POINT('Ctrl Pts',(44.8273949448428,53.6472659182591,-58.9999999999999));
#9989=CARTESIAN_POINT('Ctrl Pts',(38.4911694101435,-0.469874615149992,-146.374221095626));
#9990=CARTESIAN_POINT('Ctrl Pts',(40.9239818090476,56.7989616885694,-58.9999999999999));
#9991=CARTESIAN_POINT('Ctrl Pts',(37.3884769401616,-0.49747903844718,-152.688287840106));
#9992=CARTESIAN_POINT('Ctrl Pts',(37.,59.9327136539873,-58.9999999999999));
#9993=CARTESIAN_POINT('Ctrl Pts',(36.8261663122663,-0.524926299244587,-158.849018976011));
#9994=CARTESIAN_POINT('Ctrl Pts',(37.,59.9327136539873,-58.9999999999999));
#9995=CARTESIAN_POINT('Ctrl Pts',(63.693153039627,38.6151528517792,-59.));
#9996=CARTESIAN_POINT('Ctrl Pts',(89.4344921389827,16.4672437121532,-59.));
#9997=CARTESIAN_POINT('Ctrl Pts',(125.680065601889,4.99999999980248,-59.));
#9998=CARTESIAN_POINT('',(37.,59.9327136539873,-58.9999999999999));
#9999=CARTESIAN_POINT('Ctrl Pts',(-37.,59.9327136539873,-58.9999999999999));
#10000=CARTESIAN_POINT('Ctrl Pts',(-36.826166311831,-0.524926450656172,
-158.849019226075));
#10001=CARTESIAN_POINT('Ctrl Pts',(-40.9239818090477,56.7989616885694,-58.9999999999999));
#10002=CARTESIAN_POINT('Ctrl Pts',(-37.3884769313072,-0.49747918194178,
-152.688288074741));
#10003=CARTESIAN_POINT('Ctrl Pts',(-44.8273949448429,53.6472659182591,-58.9999999999999));
#10004=CARTESIAN_POINT('Ctrl Pts',(-38.4911693942749,-0.469874750682276,
-146.374221314448));
#10005=CARTESIAN_POINT('Ctrl Pts',(-50.7062509256847,48.9476577587424,-58.9999999999999));
#10006=CARTESIAN_POINT('Ctrl Pts',(-41.0632239464286,-0.428712779527549,
-136.886987299532));
#10007=CARTESIAN_POINT('Ctrl Pts',(-52.6698256321568,47.3857776215616,-58.9999999999999));
#10008=CARTESIAN_POINT('Ctrl Pts',(-42.0729706984543,-0.415032901765061,
-133.722571174251));
#10009=CARTESIAN_POINT('Ctrl Pts',(-56.6139853519888,44.2804710463975,-58.9999999999999));
#10010=CARTESIAN_POINT('Ctrl Pts',(-44.405954325829,-0.38783477474363,-127.432186366692));
#10011=CARTESIAN_POINT('Ctrl Pts',(-58.5945703653485,42.7370446084141,-58.9999999999999));
#10012=CARTESIAN_POINT('Ctrl Pts',(-45.7292270840355,-0.374316525484686,
-124.306271810918));
#10013=CARTESIAN_POINT('Ctrl Pts',(-62.5818489134604,39.6777872988594,-58.9999999999999));
#10014=CARTESIAN_POINT('Ctrl Pts',(-48.6902305437215,-0.347521725395707,
-118.138291319267));
#10015=CARTESIAN_POINT('Ctrl Pts',(-64.5885424482125,38.1619564272879,-58.9999999999999));
#10016=CARTESIAN_POINT('Ctrl Pts',(-50.3279822240476,-0.334245174565673,
-115.096291056904));
#10017=CARTESIAN_POINT('Ctrl Pts',(-68.6371362536135,35.1670321177717,-58.9999999999999));
#10018=CARTESIAN_POINT('Ctrl Pts',(-53.9102158131253,-0.308013841259882,
-109.142594615269));
#10019=CARTESIAN_POINT('Ctrl Pts',(-70.6790365242624,33.6879386798268,-58.9999999999999));
#10020=CARTESIAN_POINT('Ctrl Pts',(-55.8546997459087,-0.295059058784125,
-106.230970693605));
#10021=CARTESIAN_POINT('Ctrl Pts',(-74.8071420159619,30.7756311047781,-58.9999999999999));
#10022=CARTESIAN_POINT('Ctrl Pts',(-60.0336152441763,-0.269551332112253,
-100.583446484693));
#10023=CARTESIAN_POINT('Ctrl Pts',(-76.8933472370124,29.3424169676743,-58.9999999999999));
#10024=CARTESIAN_POINT('Ctrl Pts',(-62.2680277928746,-0.256998387916139,
-97.8476185470417));
#10025=CARTESIAN_POINT('Ctrl Pts',(-81.1191608440196,26.5310098615222,-58.9999999999999));
#10026=CARTESIAN_POINT('Ctrl Pts',(-67.0012120753335,-0.232374407728921,
-92.5938743445089));
#10027=CARTESIAN_POINT('Ctrl Pts',(-83.2587692299763,25.152816892474,-58.9999999999999));
#10028=CARTESIAN_POINT('Ctrl Pts',(-69.49994423464,-0.220303371737818,-90.0760234033306));
#10029=CARTESIAN_POINT('Ctrl Pts',(-87.6004873813004,22.4605939896476,-58.9999999999999));
#10030=CARTESIAN_POINT('Ctrl Pts',(-74.7282568635971,-0.196723277885987,
-85.2950967258951));
#10031=CARTESIAN_POINT('Ctrl Pts',(-89.8025971466679,21.1465640558695,-58.9999999999999));
#10032=CARTESIAN_POINT('Ctrl Pts',(-77.4577803894221,-0.18521422002526,
-83.0320726847914));
#10033=CARTESIAN_POINT('Ctrl Pts',(-94.2784162713182,18.591809090798,-58.9999999999999));
#10034=CARTESIAN_POINT('Ctrl Pts',(-83.1077052042465,-0.162838152359549,
-78.7905588175045));
#10035=CARTESIAN_POINT('Ctrl Pts',(-96.5521256306011,17.3510840595046,-58.9999999999999));
#10036=CARTESIAN_POINT('Ctrl Pts',(-86.0280376587679,-0.151971142554565,
-76.8121020841948));
#10037=CARTESIAN_POINT('Ctrl Pts',(-101.180242157587,14.952080766617,-58.9999999999999));
#10038=CARTESIAN_POINT('Ctrl Pts',(-92.0150600468664,-0.130959240925708,
-73.161088099992));
#10039=CARTESIAN_POINT('Ctrl Pts',(-103.53464932529,13.7938025050227,-58.9999999999999));
#10040=CARTESIAN_POINT('Ctrl Pts',(-95.081676134574,-0.120814349101835,
-71.4885428027475));
#10041=CARTESIAN_POINT('Ctrl Pts',(-108.33325968362,11.5688346187481,-58.9999999999999));
#10042=CARTESIAN_POINT('Ctrl Pts',(-101.314363672144,-0.101326753360565,
-68.4616401873707));
#10043=CARTESIAN_POINT('Ctrl Pts',(-110.777462874248,10.5021449940676,-58.9999999999999));
#10044=CARTESIAN_POINT('Ctrl Pts',(-104.480363396053,-0.0919840494431687,
-67.1072738889331));
#10045=CARTESIAN_POINT('Ctrl Pts',(-115.764763492932,8.469496248835,-58.9999999999999));
#10046=CARTESIAN_POINT('Ctrl Pts',(-110.864745379315,-0.0741808994402193,
-64.7198997921983));
#10047=CARTESIAN_POINT('Ctrl Pts',(-118.307860920989,7.50353712828284,-58.9999999999999));
#10048=CARTESIAN_POINT('Ctrl Pts',(-114.083064293404,-0.0657204533546665,
-63.6868647817742));
#10049=CARTESIAN_POINT('Ctrl Pts',(-123.502048229037,5.68149125852135,-58.9999999999999));
#10050=CARTESIAN_POINT('Ctrl Pts',(-120.526890365399,-0.0497618889407711,
-61.9367613594593));
#10051=CARTESIAN_POINT('Ctrl Pts',(-126.153138109028,4.82540450931203,-58.9999999999999));
#10052=CARTESIAN_POINT('Ctrl Pts',(-123.752347108032,-0.0422637706124286,
-61.2196520139871));
#10053=CARTESIAN_POINT('Ctrl Pts',(-134.282043748658,2.43566561952013,-58.9999999999999));
#10054=CARTESIAN_POINT('Ctrl Pts',(-133.377109514009,-0.0213330121512667,
-59.522904051893));
#10055=CARTESIAN_POINT('Ctrl Pts',(-139.935495507955,1.08053483677361,-58.9999999999999));
#10056=CARTESIAN_POINT('Ctrl Pts',(-139.721849114381,-0.00946396854231285,
-58.9999999999999));
#10057=CARTESIAN_POINT('Ctrl Pts',(-145.859521458148,1.99966320462804E-14,
-58.9999999999999));
#10058=CARTESIAN_POINT('Ctrl Pts',(-145.859521458148,1.99966320462804E-14,
-58.9999999999999));
#10059=CARTESIAN_POINT('Ctrl Pts',(-125.680065601889,4.99999999980248,-58.9999999999999));
#10060=CARTESIAN_POINT('Ctrl Pts',(-89.4344921389829,16.4672437121532,-58.9999999999999));
#10061=CARTESIAN_POINT('Ctrl Pts',(-63.693153039627,38.6151528517792,-58.9999999999999));
#10062=CARTESIAN_POINT('Ctrl Pts',(-37.,59.9327136539873,-58.9999999999999));
#10063=CARTESIAN_POINT('',(-36.827675631427,6.00431163122472E-14,-157.982075177761));
#10064=CARTESIAN_POINT('Ctrl Pts',(37.,59.9327136539873,-58.9999999999999));
#10065=CARTESIAN_POINT('Ctrl Pts',(36.8276756314269,6.20110919257889E-14,
-157.98207517776));
#10066=CARTESIAN_POINT('Ctrl Pts',(35.962058784555,61.0726321354551,-58.9999999999999));
#10067=CARTESIAN_POINT('Ctrl Pts',(36.6797497079439,6.26598839444921E-14,
-159.50941492147));
#10068=CARTESIAN_POINT('Ctrl Pts',(34.8494287906845,62.1881303927957,-58.9999999999999));
#10069=CARTESIAN_POINT('Ctrl Pts',(36.4288634825457,6.33418036074103E-14,
-161.114741394618));
#10070=CARTESIAN_POINT('Ctrl Pts',(32.4772932645476,64.3449801372208,-58.9999999999999));
#10071=CARTESIAN_POINT('Ctrl Pts',(35.6522781598643,6.47620449293057E-14,
-164.458171883983));
#10072=CARTESIAN_POINT('Ctrl Pts',(31.2177877322813,65.3863316243053,-58.9999999999999));
#10073=CARTESIAN_POINT('Ctrl Pts',(35.126304365244,6.55005051163517E-14,
-166.196602013066));
#10074=CARTESIAN_POINT('Ctrl Pts',(28.5544031478084,67.3695815062162,-58.9999999999999));
#10075=CARTESIAN_POINT('Ctrl Pts',(33.7243968013905,6.70122633955936E-14,
-169.755475174581));
#10076=CARTESIAN_POINT('Ctrl Pts',(27.1503938737515,68.3111074622806,-58.9999999999999));
#10077=CARTESIAN_POINT('Ctrl Pts',(32.8479279009936,6.77856653870456E-14,
-171.576162799206));
#10078=CARTESIAN_POINT('Ctrl Pts',(24.2115292157522,70.0684707648055,-58.9999999999999));
#10079=CARTESIAN_POINT('Ctrl Pts',(30.6756944321254,6.93299145588525E-14,
-175.21152369499));
#10080=CARTESIAN_POINT('Ctrl Pts',(22.6766738318099,70.8843081112658,-58.9999999999999));
#10081=CARTESIAN_POINT('Ctrl Pts',(29.3791356772816,7.01007409158914E-14,
-177.026147945389));
#10082=CARTESIAN_POINT('Ctrl Pts',(19.4899048077957,72.3648035547606,-58.9999999999999));
#10083=CARTESIAN_POINT('Ctrl Pts',(26.3232861859242,7.15849840073899E-14,
-180.520246820869));
#10084=CARTESIAN_POINT('Ctrl Pts',(17.8381180298111,73.0290133496626,-58.9999999999999));
#10085=CARTESIAN_POINT('Ctrl Pts',(24.5631346628349,7.22981500865543E-14,
-182.199131371191));
#10086=CARTESIAN_POINT('Ctrl Pts',(14.4429405853757,74.1860012886773,-58.9999999999999));
#10087=CARTESIAN_POINT('Ctrl Pts',(20.5883883156839,7.35984406902132E-14,
-185.260182463203));
#10088=CARTESIAN_POINT('Ctrl Pts',(12.6995499189248,74.6787794327899,-58.9999999999999));
#10089=CARTESIAN_POINT('Ctrl Pts',(18.3733019437226,7.41850484819666E-14,
-186.64113254965));
#10090=CARTESIAN_POINT('Ctrl Pts',(9.14636534104551,75.473548273127,-58.9999999999999));
#10091=CARTESIAN_POINT('Ctrl Pts',(13.5708791634494,7.51613194945917E-14,
-188.939399906875));
#10092=CARTESIAN_POINT('Ctrl Pts',(7.33698151150069,75.775223998754,-58.9999999999999));
#10093=CARTESIAN_POINT('Ctrl Pts',(10.9839174320015,7.55503384745273E-14,
-189.855200551742));
#10094=CARTESIAN_POINT('Ctrl Pts',(3.6851544189294,76.1798832399239,-58.9999999999999));
#10095=CARTESIAN_POINT('Ctrl Pts',(5.59736284229452,7.60764199284953E-14,
-191.093663864962));
#10096=CARTESIAN_POINT('Ctrl Pts',(1.84271115590294,76.2828667554667,-58.9999999999999));
#10097=CARTESIAN_POINT('Ctrl Pts',(2.79913386299191,7.62130211921539E-14,
-191.415240784856));
#10098=CARTESIAN_POINT('Ctrl Pts',(-1.84271115590296,76.2828667554667,-58.9999999999999));
#10099=CARTESIAN_POINT('Ctrl Pts',(-2.79913386299203,7.62130211921539E-14,
-191.415240784856));
#10100=CARTESIAN_POINT('Ctrl Pts',(-3.68515441892943,76.1798832399239,-58.9999999999999));
#10101=CARTESIAN_POINT('Ctrl Pts',(-5.59736284229463,7.60764199284953E-14,
-191.093663864962));
#10102=CARTESIAN_POINT('Ctrl Pts',(-7.33698151150072,75.775223998754,-58.9999999999999));
#10103=CARTESIAN_POINT('Ctrl Pts',(-10.9839174320017,7.55503384745273E-14,
-189.855200551742));
#10104=CARTESIAN_POINT('Ctrl Pts',(-9.14636534104554,75.473548273127,-58.9999999999999));
#10105=CARTESIAN_POINT('Ctrl Pts',(-13.5708791634495,7.51613194945917E-14,
-188.939399906875));
#10106=CARTESIAN_POINT('Ctrl Pts',(-12.6995499189249,74.6787794327899,-58.9999999999999));
#10107=CARTESIAN_POINT('Ctrl Pts',(-18.3733019437227,7.41850484819666E-14,
-186.64113254965));
#10108=CARTESIAN_POINT('Ctrl Pts',(-14.4429405853757,74.1860012886773,-58.9999999999999));
#10109=CARTESIAN_POINT('Ctrl Pts',(-20.588388315684,7.35984406902132E-14,
-185.260182463203));
#10110=CARTESIAN_POINT('Ctrl Pts',(-17.8381180298111,73.0290133496626,-58.9999999999999));
#10111=CARTESIAN_POINT('Ctrl Pts',(-24.563134662835,7.22981500865543E-14,
-182.199131371192));
#10112=CARTESIAN_POINT('Ctrl Pts',(-19.4899048077957,72.3648035547606,-58.9999999999999));
#10113=CARTESIAN_POINT('Ctrl Pts',(-26.3232861859243,7.15849840073899E-14,
-180.520246820869));
#10114=CARTESIAN_POINT('Ctrl Pts',(-22.6766738318099,70.8843081112659,-58.9999999999999));
#10115=CARTESIAN_POINT('Ctrl Pts',(-29.3791356772817,7.01007409158914E-14,
-177.026147945389));
#10116=CARTESIAN_POINT('Ctrl Pts',(-24.2115292157522,70.0684707648055,-58.9999999999999));
#10117=CARTESIAN_POINT('Ctrl Pts',(-30.6756944321255,6.93299145588525E-14,
-175.21152369499));
#10118=CARTESIAN_POINT('Ctrl Pts',(-27.1503938737515,68.3111074622807,-58.9999999999999));
#10119=CARTESIAN_POINT('Ctrl Pts',(-32.8479279009937,6.77856653870456E-14,
-171.576162799206));
#10120=CARTESIAN_POINT('Ctrl Pts',(-28.5544031478085,67.3695815062162,-58.9999999999999));
#10121=CARTESIAN_POINT('Ctrl Pts',(-33.7243968013906,6.70122633955936E-14,
-169.755475174581));
#10122=CARTESIAN_POINT('Ctrl Pts',(-31.2177877322813,65.3863316243053,-58.9999999999999));
#10123=CARTESIAN_POINT('Ctrl Pts',(-35.1263043652441,6.55005051163517E-14,
-166.196602013066));
#10124=CARTESIAN_POINT('Ctrl Pts',(-32.4772932645476,64.3449801372209,-58.9999999999999));
#10125=CARTESIAN_POINT('Ctrl Pts',(-35.6522781598644,6.47620449293057E-14,
-164.458171883983));
#10126=CARTESIAN_POINT('Ctrl Pts',(-34.8494287906845,62.1881303927957,-58.9999999999999));
#10127=CARTESIAN_POINT('Ctrl Pts',(-36.4288634825458,6.33418036074103E-14,
-161.114741394618));
#10128=CARTESIAN_POINT('Ctrl Pts',(-35.9620587845551,61.0726321354551,-58.9999999999999));
#10129=CARTESIAN_POINT('Ctrl Pts',(-36.679749707944,6.26598839444921E-14,
-159.50941492147));
#10130=CARTESIAN_POINT('Ctrl Pts',(-37.,59.9327136539873,-58.9999999999999));
#10131=CARTESIAN_POINT('Ctrl Pts',(-36.827675631427,6.20110919257889E-14,
-157.982075177761));
#10132=CARTESIAN_POINT('Ctrl Pts',(-126.333741428594,4.79470864732773,-48.9999999999999));
#10133=CARTESIAN_POINT('Ctrl Pts',(-126.333741428594,4.79470864732774,-61.));
#10134=CARTESIAN_POINT('Ctrl Pts',(-89.743409874819,16.2013907644503,-48.9999999999999));
#10135=CARTESIAN_POINT('Ctrl Pts',(-89.743409874819,16.2013907644503,-61.));
#10136=CARTESIAN_POINT('Ctrl Pts',(-63.8533409643457,38.4872243219462,-48.9999999999999));
#10137=CARTESIAN_POINT('Ctrl Pts',(-63.8533409643457,38.4872243219462,-61.));
#10138=CARTESIAN_POINT('Ctrl Pts',(-37.,59.9327136539873,-48.9999999999999));
#10139=CARTESIAN_POINT('Ctrl Pts',(-37.,59.9327136539873,-61.));
#10140=CARTESIAN_POINT('Ctrl Pts',(37.,59.9327136539873,-48.9999999999999));
#10141=CARTESIAN_POINT('Ctrl Pts',(37.,59.9327136539873,-60.9999999999999));
#10142=CARTESIAN_POINT('Ctrl Pts',(63.8533446472751,38.4872213807023,-49.));
#10143=CARTESIAN_POINT('Ctrl Pts',(63.8533446472751,38.4872213807023,-61.));
#10144=CARTESIAN_POINT('Ctrl Pts',(89.7434169764527,16.2013846514567,-49.));
#10145=CARTESIAN_POINT('Ctrl Pts',(89.7434169764527,16.2013846514567,-61.));
#10146=CARTESIAN_POINT('Ctrl Pts',(126.333756483661,4.79470395405706,-49.));
#10147=CARTESIAN_POINT('Ctrl Pts',(126.333756483661,4.79470395405707,-61.));
#10148=CARTESIAN_POINT('Origin',(-20.,72.1122755947453,-130.738895837426));
#10149=CARTESIAN_POINT('',(-20.,54.6122755947453,5.50000000000008));
#10150=CARTESIAN_POINT('Origin',(-20.,54.6122755947453,-11.9999999999999));
#10151=CARTESIAN_POINT('Origin',(-20.,54.6122755947453,-11.9999999999999));
#10152=CARTESIAN_POINT('Origin',(20.,5.00000000109418,-130.738895837426));
#10153=CARTESIAN_POINT('',(20.,54.6122755947453,-29.4999999999999));
#10154=CARTESIAN_POINT('Origin',(20.,54.6122755947453,-11.9999999999999));
#10155=CARTESIAN_POINT('Origin',(20.,54.6122755947453,-11.9999999999999));
#10156=CARTESIAN_POINT('Origin',(-45.,54.6122755947453,-11.9999999999999));
#10157=CARTESIAN_POINT('',(-45.,54.6122755947453,5.50000000000008));
#10158=CARTESIAN_POINT('',(-45.,54.6122755947453,5.50000000000008));
#10159=CARTESIAN_POINT('Origin',(-45.,54.6122755947453,-11.9999999999999));
#10160=CARTESIAN_POINT('Origin',(-45.,54.6122755947453,-11.9999999999999));
#10161=CARTESIAN_POINT('',(-45.,54.6122755947453,-25.8975067682909));
#10162=CARTESIAN_POINT('Origin',(-45.,54.6122755947453,-11.9999999999999));
#10163=CARTESIAN_POINT('Origin',(45.,54.6122755947453,-11.9999999999999));
#10164=CARTESIAN_POINT('',(45.,54.6122755947453,-29.4999999999999));
#10165=CARTESIAN_POINT('',(45.,54.6122755947453,-29.4999999999999));
#10166=CARTESIAN_POINT('Origin',(45.,54.6122755947453,-11.9999999999999));
#10167=CARTESIAN_POINT('Origin',(45.,54.6122755947453,-11.9999999999999));
#10168=CARTESIAN_POINT('Origin',(165.591979774207,54.6122755947453,-12.));
#10169=CARTESIAN_POINT('',(165.591979774207,54.6122755947453,-25.8975067682909));
#10170=CARTESIAN_POINT('Origin',(0.,89.,-11.9999999999999));
#10171=CARTESIAN_POINT('',(-2.44929359829471E-15,89.,-31.9999999999999));
#10172=CARTESIAN_POINT('Origin',(0.,89.,-11.9999999999999));
#10173=CARTESIAN_POINT('Origin',(0.,-5.00102500000001,-11.9999999999999));
#10174=CARTESIAN_POINT('',(-2.44929359829471E-15,-5.00102500000001,-31.9999999999999));
#10175=CARTESIAN_POINT('Origin',(0.,29.,-11.9999999999999));
#10176=CARTESIAN_POINT('Origin',(65.6680057154831,-5.,25.0000000000001));
#10177=CARTESIAN_POINT('Origin',(-65.6680057154831,-5.,25.0000000000001));
#10178=CARTESIAN_POINT('Origin',(-142.322386603279,-5.000025,-11.9999999999999));
#10179=CARTESIAN_POINT('',(-142.322386603279,-5.000025,-15.9999999999999));
#10180=CARTESIAN_POINT('Origin',(-115.629992744845,-5.000025,-11.9999999999999));
#10181=CARTESIAN_POINT('',(-115.629992744845,-5.000025,-27.9631510575948));
#10182=CARTESIAN_POINT('Origin',(-88.9375988864104,-5.000025,-11.9999999999999));
#10183=CARTESIAN_POINT('',(-88.9375988864104,-5.000025,-15.9999999999999));
#10184=CARTESIAN_POINT('Origin',(142.322386603279,-5.000025,-11.9999999999999));
#10185=CARTESIAN_POINT('',(142.322386603279,-5.000025,-15.9999999999999));
#10186=CARTESIAN_POINT('Origin',(115.629992744845,-5.000025,-11.9999999999999));
#10187=CARTESIAN_POINT('',(115.629992744845,-5.000025,-27.9631510575948));
#10188=CARTESIAN_POINT('Origin',(88.9375988864104,-5.000025,-11.9999999999999));
#10189=CARTESIAN_POINT('',(88.9375988864104,-5.000025,-15.9999999999999));
#14101=UNCERTAINTY_MEASURE_WITH_UNIT(LENGTH_MEASURE(0.01),#14126,
'DISTANCE_ACCURACY_VALUE',
'Maximum model space distance between geometric entities at asserted c
onnectivities');
#14112=UNCERTAINTY_MEASURE_WITH_UNIT(LENGTH_MEASURE(0.01),#14126,
'DISTANCE_ACCURACY_VALUE',
'Maximum model space distance between geometric entities at asserted c
onnectivities');
#14114=(
GEOMETRIC_REPRESENTATION_CONTEXT(3)
GLOBAL_UNCERTAINTY_ASSIGNED_CONTEXT((#14101))
GLOBAL_UNIT_ASSIGNED_CONTEXT((#14126,#14128,#14129))
REPRESENTATION_CONTEXT('','3D')
);
#14125=(
GEOMETRIC_REPRESENTATION_CONTEXT(3)
GLOBAL_UNCERTAINTY_ASSIGNED_CONTEXT((#14112))
GLOBAL_UNIT_ASSIGNED_CONTEXT((#14126,#14128,#14129))
REPRESENTATION_CONTEXT('','3D')
);
#14126=(
LENGTH_UNIT()
NAMED_UNIT(*)
SI_UNIT(.MILLI.,.METRE.)
);
#14128=(
NAMED_UNIT(*)
PLANE_ANGLE_UNIT()
SI_UNIT($,.RADIAN.)
);
#14129=(
NAMED_UNIT(*)
SI_UNIT($,.STERADIAN.)
SOLID_ANGLE_UNIT()
);
#14131=SHAPE_DEFINITION_REPRESENTATION(#14143,#14200);
#14143=PRODUCT_DEFINITION_SHAPE('',$,#14213);
#14200=SHAPE_REPRESENTATION('',(#6259),#14114);
#14211=PRODUCT_DEFINITION_CONTEXT('part definition',#14249,'design');
#14213=PRODUCT_DEFINITION('Base Plate','Base Plate',#14225,#14211);
#14225=PRODUCT_DEFINITION_FORMATION('',$,#14252);
#14249=APPLICATION_CONTEXT(
'Core Data for Automotive Mechanical Design Process');
#14250=PRODUCT_CONTEXT('part definition',#14249,'mechanical');
#14252=PRODUCT('Base Plate','Base Plate',$,(#14250));
#14263=PRESENTATION_STYLE_ASSIGNMENT((#14265));
#14265=SURFACE_STYLE_USAGE(.BOTH.,#14267);
#14267=SURFACE_SIDE_STYLE('',(#14269));
#14269=SURFACE_STYLE_FILL_AREA(#14271);
#14271=FILL_AREA_STYLE('Steel - Satin',(#14273));
#14273=FILL_AREA_STYLE_COLOUR('Steel - Satin',#14275);
#14275=COLOUR_RGB('Steel - Satin',0.627450980392157,0.627450980392157,0.627450980392157);
ENDSEC;
END-ISO-10303-21;
